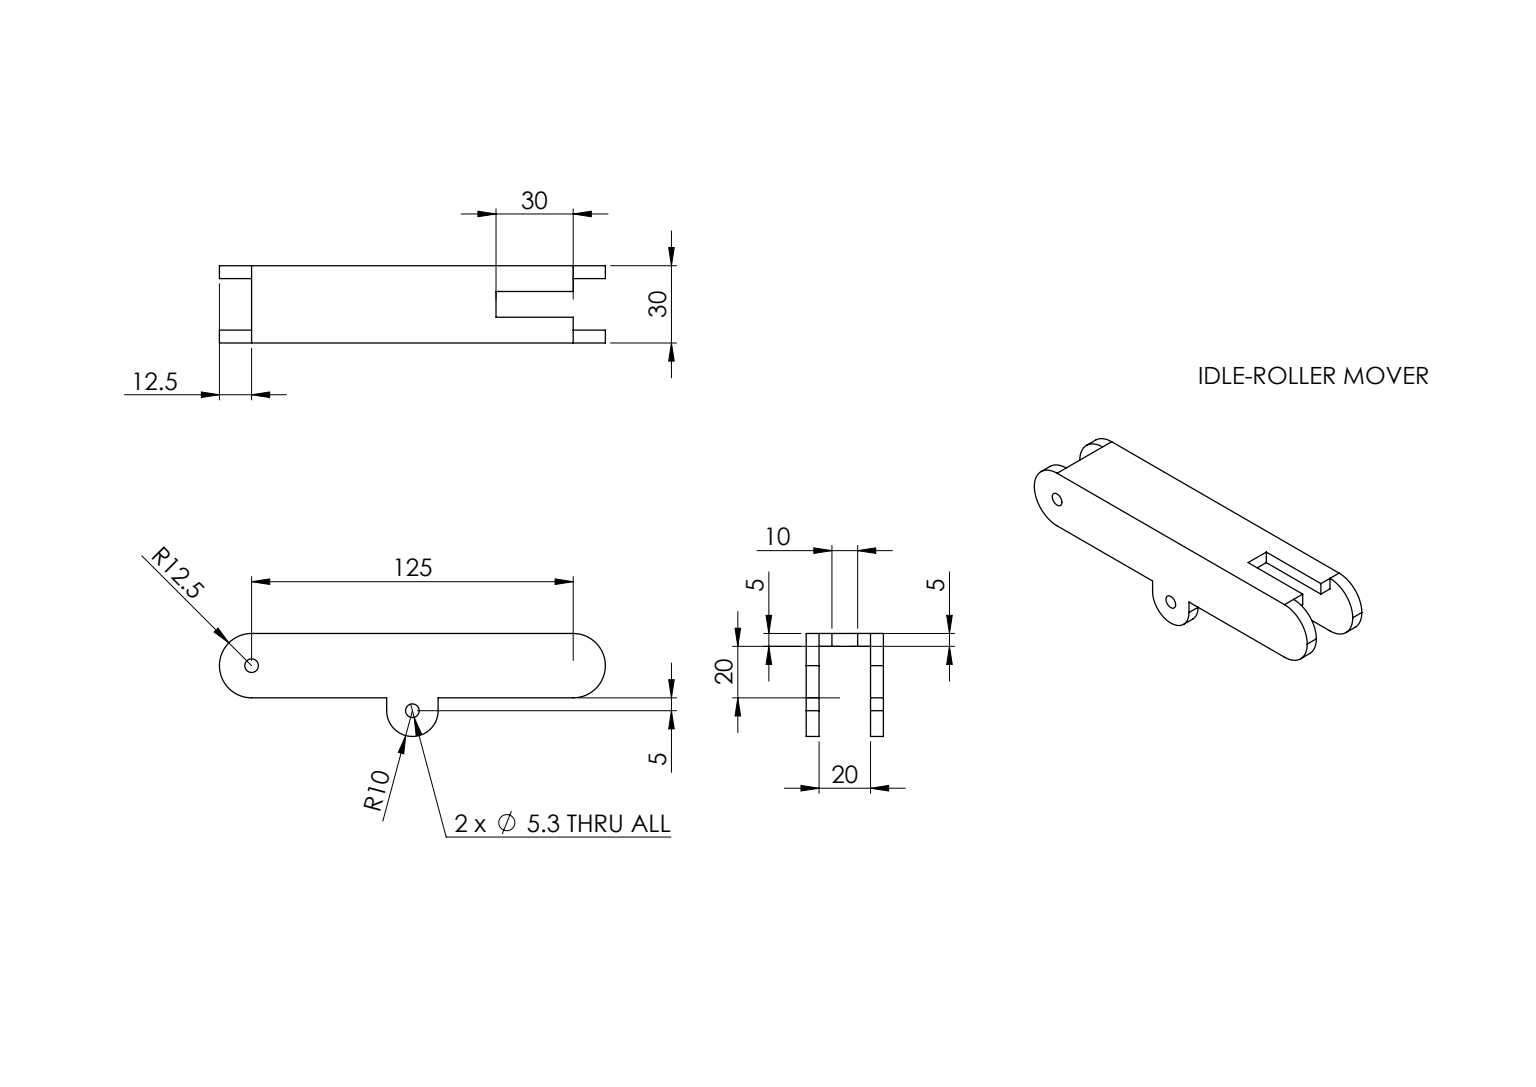
ISO-10303-21;
HEADER;
FILE_DESCRIPTION (('STEP AP214'),
    '1' );
FILE_NAME ('idle-roller mover.step',
    '2026-10-31T03:44:21',
    ( '' ),
    ( '' ),
    'SwSTEP 2.0',
    'SolidWorks 2026',
    '' );
FILE_SCHEMA (( 'AUTOMOTIVE_DESIGN' ));
ENDSEC;

DATA;
#62=VERTEX_POINT ( 'NONE', #14718 ) ;
#68=ADVANCED_FACE ( 'NONE', ( #1306 ), #2882, .T. ) ;
#78=CARTESIAN_POINT ( 'NONE',  ( -62.49999999999997158, 32.50000000000001421, 15.00000000000000000 ) ) ;
#85=LINE ( 'NONE', #5764, #17678 ) ;
#89=ORIENTED_EDGE ( 'NONE', *, *, #4960, .T. ) ;
#104=CARTESIAN_POINT ( 'NONE',  ( -62.49999999999997158, 32.50000000000001421, -15.00000000000000000 ) ) ;
#111=ORIENTED_EDGE ( 'NONE', *, *, #1854, .F. ) ;
#118=EDGE_CURVE ( 'NONE', #2113, #2665, #16595, .T. ) ;
#128=DIRECTION ( 'NONE',  ( 0.000000000000000000, -0.000000000000000000, 1.000000000000000000 ) ) ;
#164=VERTEX_POINT ( 'NONE', #8741 ) ;
#178=VERTEX_POINT ( 'NONE', #10980 ) ;
#180=ORIENTED_EDGE ( 'NONE', *, *, #9393, .F. ) ;
#211=DIRECTION ( 'NONE',  ( -0.000000000000000000, -0.000000000000000000, 1.000000000000000000 ) ) ;
#227=DIRECTION ( 'NONE',  ( 0.000000000000000000, -0.000000000000000000, 1.000000000000000000 ) ) ;
#232=EDGE_LOOP ( 'NONE', ( #13470, #855 ) ) ;
#236=PLANE ( 'NONE',  #7905 ) ;
#241=AXIS2_PLACEMENT_3D ( 'NONE', #17266, #3826, #15783 ) ;
#248=VERTEX_POINT ( 'NONE', #13911 ) ;
#260=CARTESIAN_POINT ( 'NONE',  ( 9.999999999999994671, 20.00000000000001421, -9.999999999999998224 ) ) ;
#273=VERTEX_POINT ( 'NONE', #10784 ) ;
#285=AXIS2_PLACEMENT_3D ( 'NONE', #12614, #3232, #18241 ) ;
#291=DIRECTION ( 'NONE',  ( 1.000000000000000000, 0.000000000000000000, 0.000000000000000000 ) ) ;
#304=FILL_AREA_STYLE_COLOUR ( '', #11512 ) ;
#308=CIRCLE ( 'NONE', #3740, 12.49999999999999645 ) ;
#311=DIRECTION ( 'NONE',  ( 1.000000000000000000, -0.000000000000000000, 0.000000000000000000 ) ) ;
#322=DIRECTION ( 'NONE',  ( 0.000000000000000000, 0.000000000000000000, -1.000000000000000000 ) ) ;
#342=FACE_OUTER_BOUND ( 'NONE', #4754, .T. ) ;
#350=AXIS2_PLACEMENT_3D ( 'NONE', #1219, #5627, #11312 ) ;
#355=DIRECTION ( 'NONE',  ( 0.000000000000000000, 0.000000000000000000, -1.000000000000000000 ) ) ;
#364=AXIS2_PLACEMENT_3D ( 'NONE', #11139, #15465, #17247 ) ;
#397=ORIENTED_EDGE ( 'NONE', *, *, #12870, .T. ) ;
#409=PLANE ( 'NONE',  #5457 ) ;
#418=AXIS2_PLACEMENT_3D ( 'NONE', #11692, #1217, #13364 ) ;
#474=DIRECTION ( 'NONE',  ( 0.000000000000000000, -0.000000000000000000, 1.000000000000000000 ) ) ;
#485=EDGE_LOOP ( 'NONE', ( #9928, #11888, #6922, #5916 ) ) ;
#487=SURFACE_SIDE_STYLE ('',( #18064 ) ) ;
#533=ORIENTED_EDGE ( 'NONE', *, *, #13929, .T. ) ;
#534=EDGE_CURVE ( 'NONE', #17889, #2561, #18649, .T. ) ;
#536=EDGE_CURVE ( 'NONE', #9835, #14591, #15254, .T. ) ;
#540=EDGE_CURVE ( 'NONE', #178, #11648, #7706, .T. ) ;
#563=ORIENTED_EDGE ( 'NONE', *, *, #9312, .F. ) ;
#574=STYLED_ITEM('',(#19461),#14815);
#579=MECHANICAL_DESIGN_GEOMETRIC_PRESENTATION_REPRESENTATION('',(#14012),#4333);
#599=VECTOR ( 'NONE', #11017, 1000.000000000000000 ) ;
#642=CIRCLE ( 'NONE', #6581, 9.999999999999998224 ) ;
#659=SHAPE_REPRESENTATION ( 'idle-roller mover', ( #10359 ), #7771 ) ;
#671=VERTEX_POINT ( 'NONE', #6520 ) ;
#674=FACE_OUTER_BOUND ( 'NONE', #12815, .T. ) ;
#680=CIRCLE ( 'NONE', #11624, 12.49999999999999645 ) ;
#699=PLANE ( 'NONE',  #16848 ) ;
#711=CYLINDRICAL_SURFACE ( 'NONE', #16596, 12.49999999999999645 ) ;
#768=CARTESIAN_POINT ( 'NONE',  ( 10.00000000000000000, 0.000000000000000000, 9.999999999999998224 ) ) ;
#770=DIRECTION ( 'NONE',  ( -0.000000000000000000, -0.000000000000000000, 1.000000000000000000 ) ) ;
#804=VECTOR ( 'NONE', #311, 1000.000000000000000 ) ;
#813=EDGE_CURVE ( 'NONE', #7075, #6422, #11344, .T. ) ;
#835=ORIENTED_EDGE ( 'NONE', *, *, #16599, .T. ) ;
#846=AXIS2_PLACEMENT_3D ( 'NONE', #4289, #19020, #14574 ) ;
#851=ORIENTED_EDGE ( 'NONE', *, *, #8320, .T. ) ;
#854=EDGE_LOOP ( 'NONE', ( #10763, #14737 ) ) ;
#855=ORIENTED_EDGE ( 'NONE', *, *, #534, .T. ) ;
#903=ADVANCED_FACE ( 'NONE', ( #342 ), #236, .F. ) ;
#904=DIRECTION ( 'NONE',  ( 1.000000000000000000, 0.000000000000000000, 0.000000000000000000 ) ) ;
#916=DIRECTION ( 'NONE',  ( -0.000000000000000000, 0.000000000000000000, -1.000000000000000000 ) ) ;
#933=VECTOR ( 'NONE', #904, 1000.000000000000000 ) ;
#946=CARTESIAN_POINT ( 'NONE',  ( -9.999999999999998224, 15.00000000000001776, -9.999999999999998224 ) ) ;
#969=LINE ( 'NONE', #768, #15487 ) ;
#970=CARTESIAN_POINT ( 'NONE',  ( 1.925929944387235853E-31, 15.00000000000001599, 9.999999999999998224 ) ) ;
#980=FACE_OUTER_BOUND ( 'NONE', #485, .T. ) ;
#981=LINE ( 'NONE', #18936, #3407 ) ;
#985=EDGE_LOOP ( 'NONE', ( #10470, #4595, #111, #14625 ) ) ;
#992=DIRECTION ( 'NONE',  ( 0.000000000000000000, 1.000000000000000000, 0.000000000000000000 ) ) ;
#1012=LINE ( 'NONE', #8840, #1882 ) ;
#1015=FACE_OUTER_BOUND ( 'NONE', #18810, .T. ) ;
#1027=ORIENTED_EDGE ( 'NONE', *, *, #13929, .F. ) ;
#1062=CARTESIAN_POINT ( 'NONE',  ( 32.49999999999998579, 40.00000000000001421, 15.00000000000000000 ) ) ;
#1103=DIRECTION ( 'NONE',  ( 0.000000000000000000, 0.000000000000000000, -1.000000000000000000 ) ) ;
#1116=ORIENTED_EDGE ( 'NONE', *, *, #536, .T. ) ;
#1125=DIRECTION ( 'NONE',  ( -0.000000000000000000, -0.000000000000000000, 1.000000000000000000 ) ) ;
#1149=ORIENTED_EDGE ( 'NONE', *, *, #15610, .T. ) ;
#1184=DIRECTION ( 'NONE',  ( 1.000000000000000000, 0.000000000000000000, 0.000000000000000000 ) ) ;
#1203=DIRECTION ( 'NONE',  ( 0.000000000000000000, 0.000000000000000000, -1.000000000000000000 ) ) ;
#1217=DIRECTION ( 'NONE',  ( 0.000000000000000000, 1.000000000000000000, 0.000000000000000000 ) ) ;
#1219=CARTESIAN_POINT ( 'NONE',  ( -62.49999999999997158, 32.50000000000001421, -9.999999999999998224 ) ) ;
#1239=ORIENTED_EDGE ( 'NONE', *, *, #7238, .T. ) ;
#1247=VERTEX_POINT ( 'NONE', #18585 ) ;
#1281=CARTESIAN_POINT ( 'NONE',  ( -62.49999999999997158, 32.50000000000001421, 9.999999999999998224 ) ) ;
#1298=ORIENTED_EDGE ( 'NONE', *, *, #536, .F. ) ;
#1303=AXIS2_PLACEMENT_3D ( 'NONE', #18296, #7784, #10909 ) ;
#1306=FACE_OUTER_BOUND ( 'NONE', #16945, .T. ) ;
#1315=VECTOR ( 'NONE', #1680, 1000.000000000000000 ) ;
#1349=CARTESIAN_POINT ( 'NONE',  ( -62.49999999999997158, 20.00000000000001421, -15.00000000000000000 ) ) ;
#1351=LINE ( 'NONE', #1062, #18417 ) ;
#1353=CARTESIAN_POINT ( 'NONE',  ( 32.49999999999998579, 45.00000000000001421, 5.000000000000003553 ) ) ;
#1359=PRODUCT_DEFINITION ( 'UNKNOWN', '', #1975, #10856 ) ;
#1381=VECTOR ( 'NONE', #19322, 1000.000000000000000 ) ;
#1404=CARTESIAN_POINT ( 'NONE',  ( -74.99999999999997158, 32.50000000000001421, -15.00000000000000000 ) ) ;
#1452=CARTESIAN_POINT ( 'NONE',  ( 32.49999999999998579, 5.000000000000018652, -4.999999999999996447 ) ) ;
#1457=FACE_OUTER_BOUND ( 'NONE', #9301, .T. ) ;
#1462=VERTEX_POINT ( 'NONE', #18073 ) ;
#1485=CARTESIAN_POINT ( 'NONE',  ( -62.49999999999997158, 32.50000000000001421, -15.00000000000000000 ) ) ;
#1487=DIRECTION ( 'NONE',  ( 1.000000000000000000, 0.000000000000000000, 0.000000000000000000 ) ) ;
#1488=ADVANCED_FACE ( 'NONE', ( #2972 ), #16696, .T. ) ;
#1518=VECTOR ( 'NONE', #17948, 1000.000000000000000 ) ;
#1530=DIRECTION ( 'NONE',  ( 0.000000000000000000, 0.000000000000000000, -1.000000000000000000 ) ) ;
#1567=AXIS2_PLACEMENT_3D ( 'NONE', #6482, #12664, #14320 ) ;
#1594=AXIS2_PLACEMENT_3D ( 'NONE', #7740, #4809, #4899 ) ;
#1613=ADVANCED_FACE ( 'NONE', ( #13831 ), #12652, .F. ) ;
#1614=EDGE_CURVE ( 'NONE', #10922, #10528, #6471, .T. ) ;
#1617=DIRECTION ( 'NONE',  ( 0.000000000000000000, 0.000000000000000000, -1.000000000000000000 ) ) ;
#1618=ADVANCED_FACE ( 'NONE', ( #9596, #12451, #10883 ), #2072, .F. ) ;
#1621=CARTESIAN_POINT ( 'NONE',  ( -62.49999999999997158, 20.00000000000001421, -15.00000000000000000 ) ) ;
#1623=FACE_OUTER_BOUND ( 'NONE', #18650, .T. ) ;
#1674=ORIENTED_EDGE ( 'NONE', *, *, #15749, .F. ) ;
#1680=DIRECTION ( 'NONE',  ( 1.000000000000000000, -0.000000000000000000, 0.000000000000000000 ) ) ;
#1682=DIRECTION ( 'NONE',  ( -0.000000000000000000, -0.000000000000000000, 1.000000000000000000 ) ) ;
#1705=ORIENTED_EDGE ( 'NONE', *, *, #3062, .F. ) ;
#1721=ADVANCED_FACE ( 'NONE', ( #15306 ), #699, .F. ) ;
#1724=ORIENTED_EDGE ( 'NONE', *, *, #17366, .F. ) ;
#1739=CYLINDRICAL_SURFACE ( 'NONE', #17926, 12.49999999999999645 ) ;
#1780=EDGE_CURVE ( 'NONE', #9457, #2897, #16089, .T. ) ;
#1825=CARTESIAN_POINT ( 'NONE',  ( 62.49999999999998579, 45.00000000000001421, -9.999999999999998224 ) ) ;
#1854=EDGE_CURVE ( 'NONE', #7017, #7129, #17757, .T. ) ;
#1882=VECTOR ( 'NONE', #5606, 1000.000000000000000 ) ;
#1900=CIRCLE ( 'NONE', #12847, 12.49999999999999645 ) ;
#1955=ORIENTED_EDGE ( 'NONE', *, *, #11365, .T. ) ;
#1970=EDGE_CURVE ( 'NONE', #17741, #6607, #4613, .T. ) ;
#1975=PRODUCT_DEFINITION_FORMATION_WITH_SPECIFIED_SOURCE ( 'ANY', '', #10075, .NOT_KNOWN. ) ;
#2016=LINE ( 'NONE', #10822, #5296 ) ;
#2022=ORIENTED_EDGE ( 'NONE', *, *, #11676, .F. ) ;
#2028=CARTESIAN_POINT ( 'NONE',  ( 0.000000000000000000, 20.00000000000001421, -9.999999999999998224 ) ) ;
#2042=CYLINDRICAL_SURFACE ( 'NONE', #285, 2.649999999999988365 ) ;
#2071=LINE ( 'NONE', #16695, #13282 ) ;
#2072=PLANE ( 'NONE',  #12758 ) ;
#2079=DIRECTION ( 'NONE',  ( -1.000000000000000000, 0.000000000000000000, 1.224646799147353207E-16 ) ) ;
#2103=LINE ( 'NONE', #15724, #17590 ) ;
#2112=DIRECTION ( 'NONE',  ( -0.000000000000000000, 1.000000000000000000, -0.000000000000000000 ) ) ;
#2113=VERTEX_POINT ( 'NONE', #13896 ) ;
#2121=CIRCLE ( 'NONE', #8046, 2.649999999999985700 ) ;
#2133=ORIENTED_EDGE ( 'NONE', *, *, #13598, .F. ) ;
#2134=FACE_OUTER_BOUND ( 'NONE', #12540, .T. ) ;
#2136=VECTOR ( 'NONE', #2285, 1000.000000000000000 ) ;
#2137=EDGE_CURVE ( 'NONE', #3410, #5817, #10817, .T. ) ;
#2143=ORIENTED_EDGE ( 'NONE', *, *, #17441, .F. ) ;
#2192=VERTEX_POINT ( 'NONE', #14487 ) ;
#2213=DIRECTION ( 'NONE',  ( 0.000000000000000000, 0.000000000000000000, -1.000000000000000000 ) ) ;
#2214=ORIENTED_EDGE ( 'NONE', *, *, #15651, .T. ) ;
#2217=EDGE_CURVE ( 'NONE', #62, #18826, #7388, .T. ) ;
#2230=ADVANCED_FACE ( 'NONE', ( #13018 ), #14284, .T. ) ;
#2240=ORIENTED_EDGE ( 'NONE', *, *, #11403, .T. ) ;
#2272=DIRECTION ( 'NONE',  ( -0.000000000000000000, -0.000000000000000000, -1.000000000000000000 ) ) ;
#2285=DIRECTION ( 'NONE',  ( -0.000000000000000000, -0.000000000000000000, -1.000000000000000000 ) ) ;
#2311=ORIENTED_EDGE ( 'NONE', *, *, #1970, .T. ) ;
#2356=DIRECTION ( 'NONE',  ( 1.000000000000000000, 0.000000000000000000, 0.000000000000000000 ) ) ;
#2358=ORIENTED_EDGE ( 'NONE', *, *, #6658, .T. ) ;
#2373=CARTESIAN_POINT ( 'NONE',  ( 2.649999999999987477, 15.00000000000001599, 15.00000000000000178 ) ) ;
#2377=CARTESIAN_POINT ( 'NONE',  ( 10.00000000000000000, 15.00000000000001776, 15.00000000000000000 ) ) ;
#2414=VECTOR ( 'NONE', #13659, 1000.000000000000000 ) ;
#2433=VERTEX_POINT ( 'NONE', #3860 ) ;
#2437=VECTOR ( 'NONE', #17878, 1000.000000000000000 ) ;
#2454=EDGE_CURVE ( 'NONE', #2113, #6630, #5693, .T. ) ;
#2457=ORIENTED_EDGE ( 'NONE', *, *, #3348, .T. ) ;
#2459=DIRECTION ( 'NONE',  ( -0.000000000000000000, -0.000000000000000000, 1.000000000000000000 ) ) ;
#2548=CIRCLE ( 'NONE', #17575, 12.49999999999999645 ) ;
#2559=AXIS2_PLACEMENT_3D ( 'NONE', #1281, #8422, #19338 ) ;
#2561=VERTEX_POINT ( 'NONE', #17689 ) ;
#2587=LINE ( 'NONE', #14415, #2136 ) ;
#2620=CARTESIAN_POINT ( 'NONE',  ( 75.00000000000000000, 32.50000000000001421, 15.00000000000000000 ) ) ;
#2633=ADVANCED_FACE ( 'NONE', ( #8354 ), #5512, .T. ) ;
#2642=ORIENTED_EDGE ( 'NONE', *, *, #118, .F. ) ;
#2646=CARTESIAN_POINT ( 'NONE',  ( -62.49999999999997158, 32.50000000000001421, 15.00000000000000000 ) ) ;
#2665=VERTEX_POINT ( 'NONE', #1404 ) ;
#2685=DIRECTION ( 'NONE',  ( 1.000000000000000000, 0.000000000000000000, -0.000000000000000000 ) ) ;
#2723=EDGE_CURVE ( 'NONE', #1247, #2192, #18742, .T. ) ;
#2725=DIRECTION ( 'NONE',  ( -1.000000000000000000, 0.000000000000000000, 1.224646799147353207E-16 ) ) ;
#2802=VERTEX_POINT ( 'NONE', #12743 ) ;
#2812=CIRCLE ( 'NONE', #13129, 12.49999999999999645 ) ;
#2814=AXIS2_PLACEMENT_3D ( 'NONE', #12299, #355, #16535 ) ;
#2825=EDGE_CURVE ( 'NONE', #8729, #6112, #16066, .T. ) ;
#2830=ORIENTED_EDGE ( 'NONE', *, *, #4507, .T. ) ;
#2859=AXIS2_PLACEMENT_3D ( 'NONE', #19237, #5483, #7155 ) ;
#2871=CARTESIAN_POINT ( 'NONE',  ( 0.000000000000000000, 0.000000000000000000, 0.000000000000000000 ) ) ;
#2882=CYLINDRICAL_SURFACE ( 'NONE', #11472, 12.49999999999999645 ) ;
#2895=EDGE_LOOP ( 'NONE', ( #13031, #2901 ) ) ;
#2897=VERTEX_POINT ( 'NONE', #260 ) ;
#2901=ORIENTED_EDGE ( 'NONE', *, *, #17364, .F. ) ;
#2913=AXIS2_PLACEMENT_3D ( 'NONE', #17621, #11508, #17325 ) ;
#2914=ORIENTED_EDGE ( 'NONE', *, *, #9264, .T. ) ;
#2922=ORIENTED_EDGE ( 'NONE', *, *, #15885, .T. ) ;
#2932=CARTESIAN_POINT ( 'NONE',  ( 75.00000000000000000, 32.50000000000001421, -15.00000000000000000 ) ) ;
#2933=ORIENTED_EDGE ( 'NONE', *, *, #11365, .F. ) ;
#2937=CARTESIAN_POINT ( 'NONE',  ( 62.49999999999998579, 45.00000000000001421, 9.999999999999998224 ) ) ;
#2957=EDGE_CURVE ( 'NONE', #2433, #6630, #8982, .T. ) ;
#2967=VECTOR ( 'NONE', #17100, 1000.000000000000000 ) ;
#2972=FACE_OUTER_BOUND ( 'NONE', #17073, .T. ) ;
#2981=ORIENTED_EDGE ( 'NONE', *, *, #7617, .T. ) ;
#2982=ADVANCED_FACE ( 'NONE', ( #15072 ), #1739, .T. ) ;
#3012=ORIENTED_EDGE ( 'NONE', *, *, #6302, .F. ) ;
#3055=EDGE_CURVE ( 'NONE', #19088, #6925, #8275, .T. ) ;
#3062=EDGE_CURVE ( 'NONE', #10814, #11786, #3397, .T. ) ;
#3066=DIRECTION ( 'NONE',  ( 1.000000000000000000, -0.000000000000000000, 0.000000000000000000 ) ) ;
#3077=CARTESIAN_POINT ( 'NONE',  ( -62.49999999999997158, 32.50000000000001421, -15.00000000000000000 ) ) ;
#3090=DIRECTION ( 'NONE',  ( 1.000000000000000000, 0.000000000000000000, 0.000000000000000000 ) ) ;
#3140=CIRCLE ( 'NONE', #16292, 2.649999999999987477 ) ;
#3158=CARTESIAN_POINT ( 'NONE',  ( -2.649999999999987477, 15.00000000000001599, 15.00000000000000178 ) ) ;
#3164=DIRECTION ( 'NONE',  ( 1.000000000000000000, 0.000000000000000000, 0.000000000000000000 ) ) ;
#3170=AXIS2_PLACEMENT_3D ( 'NONE', #18983, #12788, #8571 ) ;
#3192=CARTESIAN_POINT ( 'NONE',  ( -62.49999999999997158, 45.00000000000001421, 15.00000000000000000 ) ) ;
#3193=LINE ( 'NONE', #5830, #8882 ) ;
#3232=DIRECTION ( 'NONE',  ( -0.000000000000000000, -0.000000000000000000, 1.000000000000000000 ) ) ;
#3256=CARTESIAN_POINT ( 'NONE',  ( 62.49999999999998579, 40.00000000000001421, 9.999999999999998224 ) ) ;
#3272=ORIENTED_EDGE ( 'NONE', *, *, #10957, .T. ) ;
#3287=ORIENTED_EDGE ( 'NONE', *, *, #17366, .T. ) ;
#3294=CARTESIAN_POINT ( 'NONE',  ( 32.49999999999998579, 5.000000000000018652, 5.000000000000003553 ) ) ;
#3307=EDGE_CURVE ( 'NONE', #5263, #6112, #12645, .T. ) ;
#3322=LINE ( 'NONE', #3602, #15614 ) ;
#3323=ORIENTED_EDGE ( 'NONE', *, *, #17364, .T. ) ;
#3328=ORIENTED_EDGE ( 'NONE', *, *, #12262, .F. ) ;
#3337=DIRECTION ( 'NONE',  ( -0.000000000000000000, -0.000000000000000000, 1.000000000000000000 ) ) ;
#3342=ORIENTED_EDGE ( 'NONE', *, *, #17496, .T. ) ;
#3343=( NAMED_UNIT ( * ) PLANE_ANGLE_UNIT ( ) SI_UNIT ( $, .RADIAN. ) );
#3348=EDGE_CURVE ( 'NONE', #7873, #4201, #3193, .T. ) ;
#3355=DIRECTION ( 'NONE',  ( 0.000000000000000000, 0.000000000000000000, -1.000000000000000000 ) ) ;
#3381=FACE_OUTER_BOUND ( 'NONE', #7891, .T. ) ;
#3386=DIRECTION ( 'NONE',  ( -0.000000000000000000, -0.000000000000000000, 1.000000000000000000 ) ) ;
#3397=LINE ( 'NONE', #2028, #17988 ) ;
#3407=VECTOR ( 'NONE', #11356, 1000.000000000000000 ) ;
#3410=VERTEX_POINT ( 'NONE', #9155 ) ;
#3437=ORIENTED_EDGE ( 'NONE', *, *, #2137, .T. ) ;
#3441=ORIENTED_EDGE ( 'NONE', *, *, #6041, .T. ) ;
#3452=DIRECTION ( 'NONE',  ( 0.000000000000000000, 0.000000000000000000, 1.000000000000000000 ) ) ;
#3465=CIRCLE ( 'NONE', #4729, 2.649999999999988809 ) ;
#3482=LINE ( 'NONE', #7972, #7826 ) ;
#3506=CARTESIAN_POINT ( 'NONE',  ( 75.00000000000000000, 32.50000000000001421, 15.00000000000000000 ) ) ;
#3509=DIRECTION ( 'NONE',  ( 0.000000000000000000, 0.000000000000000000, -1.000000000000000000 ) ) ;
#3516=DIRECTION ( 'NONE',  ( -0.000000000000000000, 0.000000000000000000, -1.000000000000000000 ) ) ;
#3527=ORIENTED_EDGE ( 'NONE', *, *, #2217, .F. ) ;
#3554=CARTESIAN_POINT ( 'NONE',  ( 62.50000000000000000, 32.50000000000001421, 15.00000000000000000 ) ) ;
#3565=CARTESIAN_POINT ( 'NONE',  ( 62.49999999999998579, 45.00000000000001421, 15.00000000000000000 ) ) ;
#3582=EDGE_CURVE ( 'NONE', #15125, #273, #11092, .T. ) ;
#3586=ORIENTED_EDGE ( 'NONE', *, *, #4960, .F. ) ;
#3602=CARTESIAN_POINT ( 'NONE',  ( 9.999999999999994671, 20.00000000000001421, 15.00000000000000000 ) ) ;
#3613=LINE ( 'NONE', #7829, #15804 ) ;
#3644=DIRECTION ( 'NONE',  ( -0.000000000000000000, -0.000000000000000000, 1.000000000000000000 ) ) ;
#3648=EDGE_CURVE ( 'NONE', #10516, #8542, #18674, .T. ) ;
#3659=ADVANCED_FACE ( 'NONE', ( #16110, #18872, #1015 ), #10200, .F. ) ;
#3673=CARTESIAN_POINT ( 'NONE',  ( -62.49999999999997158, 32.50000000000001421, 15.00000000000000000 ) ) ;
#3675=DIRECTION ( 'NONE',  ( -0.000000000000000000, -0.000000000000000000, 1.000000000000000000 ) ) ;
#3700=AXIS2_PLACEMENT_3D ( 'NONE', #12562, #3644, #18372 ) ;
#3705=CARTESIAN_POINT ( 'NONE',  ( 62.49999999999998579, 20.00000000000001421, 15.00000000000000000 ) ) ;
#3708=VERTEX_POINT ( 'NONE', #12869 ) ;
#3715=DIRECTION ( 'NONE',  ( -1.224646799147353207E-16, 0.000000000000000000, -1.000000000000000000 ) ) ;
#3740=AXIS2_PLACEMENT_3D ( 'NONE', #11015, #2213, #17022 ) ;
#3763=CARTESIAN_POINT ( 'NONE',  ( 1.925929944387235853E-31, 15.00000000000001599, 15.00000000000000000 ) ) ;
#3771=VERTEX_POINT ( 'NONE', #19172 ) ;
#3774=ADVANCED_FACE ( 'NONE', ( #17297 ), #9815, .T. ) ;
#3796=DIRECTION ( 'NONE',  ( -1.000000000000000000, 0.000000000000000000, 0.000000000000000000 ) ) ;
#3799=ORIENTED_EDGE ( 'NONE', *, *, #16660, .T. ) ;
#3800=DIRECTION ( 'NONE',  ( -1.000000000000000000, 0.000000000000000000, -0.000000000000000000 ) ) ;
#3818=DIRECTION ( 'NONE',  ( 1.000000000000000000, 0.000000000000000000, 0.000000000000000000 ) ) ;
#3826=DIRECTION ( 'NONE',  ( -0.000000000000000000, -0.000000000000000000, 1.000000000000000000 ) ) ;
#3860=CARTESIAN_POINT ( 'NONE',  ( -62.49999999999997158, 40.00000000000001421, -9.999999999999998224 ) ) ;
#3896=EDGE_LOOP ( 'NONE', ( #7677, #3272, #11341, #7131 ) ) ;
#3907=EDGE_LOOP ( 'NONE', ( #12635, #19029, #3342, #11438 ) ) ;
#3914=LINE ( 'NONE', #8307, #7534 ) ;
#3939=LINE ( 'NONE', #17477, #5569 ) ;
#3959=FACE_OUTER_BOUND ( 'NONE', #13204, .T. ) ;
#3989=ORIENTED_EDGE ( 'NONE', *, *, #540, .T. ) ;
#3993=ORIENTED_EDGE ( 'NONE', *, *, #9285, .F. ) ;
#4003=ADVANCED_FACE ( 'NONE', ( #4635 ), #409, .F. ) ;
#4013=LINE ( 'NONE', #15216, #14946 ) ;
#4028=LINE ( 'NONE', #9891, #9519 ) ;
#4036=DIRECTION ( 'NONE',  ( -0.000000000000000000, 0.000000000000000000, -1.000000000000000000 ) ) ;
#4070=ORIENTED_EDGE ( 'NONE', *, *, #7617, .F. ) ;
#4083=CARTESIAN_POINT ( 'NONE',  ( 1.925929944387235853E-31, 15.00000000000001599, -9.999999999999998224 ) ) ;
#4086=ORIENTED_EDGE ( 'NONE', *, *, #7359, .F. ) ;
#4102=CARTESIAN_POINT ( 'NONE',  ( -9.999999999999996447, 25.00000000000001776, 15.00000000000000000 ) ) ;
#4133=EDGE_CURVE ( 'NONE', #13670, #1462, #2071, .T. ) ;
#4136=( NAMED_UNIT ( * ) PLANE_ANGLE_UNIT ( ) SI_UNIT ( $, .RADIAN. ) );
#4139=ORIENTED_EDGE ( 'NONE', *, *, #5848, .T. ) ;
#4162=FACE_OUTER_BOUND ( 'NONE', #4530, .T. ) ;
#4163=ORIENTED_EDGE ( 'NONE', *, *, #6041, .F. ) ;
#4179=VERTEX_POINT ( 'NONE', #9797 ) ;
#4195=PLANE ( 'NONE',  #6785 ) ;
#4201=VERTEX_POINT ( 'NONE', #15890 ) ;
#4237=EDGE_CURVE ( 'NONE', #248, #17308, #4028, .T. ) ;
#4247=ADVANCED_FACE ( 'NONE', ( #11558 ), #11458, .F. ) ;
#4248=VERTEX_POINT ( 'NONE', #2373 ) ;
#4262=CARTESIAN_POINT ( 'NONE',  ( 62.50000000000000000, 32.50000000000001421, -9.999999999999998224 ) ) ;
#4280=ORIENTED_EDGE ( 'NONE', *, *, #18031, .F. ) ;
#4289=CARTESIAN_POINT ( 'NONE',  ( -62.49999999999997158, 32.50000000000001421, 15.00000000000000000 ) ) ;
#4333=( GEOMETRIC_REPRESENTATION_CONTEXT ( 3 ) GLOBAL_UNCERTAINTY_ASSIGNED_CONTEXT ( ( #7345 ) ) GLOBAL_UNIT_ASSIGNED_CONTEXT ( ( #10583, #15004, #13903 ) ) REPRESENTATION_CONTEXT ( 'NONE', 'WORKASPACE' ) );
#4358=LINE ( 'NONE', #3192, #4605 ) ;
#4377=DIRECTION ( 'NONE',  ( -1.000000000000000000, 0.000000000000000000, 0.000000000000000000 ) ) ;
#4388=CIRCLE ( 'NONE', #14066, 12.49999999999999645 ) ;
#4393=DIRECTION ( 'NONE',  ( -0.000000000000000000, 0.000000000000000000, -1.000000000000000000 ) ) ;
#4438=CIRCLE ( 'NONE', #16334, 2.649999999999985700 ) ;
#4463=DIRECTION ( 'NONE',  ( -0.000000000000000000, -0.000000000000000000, 1.000000000000000000 ) ) ;
#4477=EDGE_CURVE ( 'NONE', #10516, #7873, #13293, .T. ) ;
#4487=CARTESIAN_POINT ( 'NONE',  ( 2.649999999999988365, 15.00000000000001599, 15.00000000000000000 ) ) ;
#4497=DIRECTION ( 'NONE',  ( 0.000000000000000000, 0.000000000000000000, -1.000000000000000000 ) ) ;
#4501=ORIENTED_EDGE ( 'NONE', *, *, #2957, .F. ) ;
#4502=ORIENTED_EDGE ( 'NONE', *, *, #18699, .T. ) ;
#4507=EDGE_CURVE ( 'NONE', #1247, #17702, #3613, .T. ) ;
#4513=VERTEX_POINT ( 'NONE', #6449 ) ;
#4530=EDGE_LOOP ( 'NONE', ( #7481, #5283, #8817, #3012 ) ) ;
#4532=AXIS2_PLACEMENT_3D ( 'NONE', #15814, #6878, #17392 ) ;
#4555=ORIENTED_EDGE ( 'NONE', *, *, #2825, .T. ) ;
#4568=FACE_OUTER_BOUND ( 'NONE', #16154, .T. ) ;
#4587=VECTOR ( 'NONE', #16481, 1000.000000000000000 ) ;
#4595=ORIENTED_EDGE ( 'NONE', *, *, #10584, .T. ) ;
#4605=VECTOR ( 'NONE', #4463, 1000.000000000000000 ) ;
#4608=CARTESIAN_POINT ( 'NONE',  ( -59.84999999999998721, 32.50000000000001421, -15.00000000000000000 ) ) ;
#4613=LINE ( 'NONE', #13324, #19332 ) ;
#4623=PRESENTATION_STYLE_ASSIGNMENT (( #18355 ) ) ;
#4628=DIRECTION ( 'NONE',  ( 1.000000000000000000, 0.000000000000000000, -0.000000000000000000 ) ) ;
#4635=FACE_OUTER_BOUND ( 'NONE', #19090, .T. ) ;
#4644=FACE_OUTER_BOUND ( 'NONE', #10586, .T. ) ;
#4649=ORIENTED_EDGE ( 'NONE', *, *, #14215, .F. ) ;
#4673=AXIS2_PLACEMENT_3D ( 'NONE', #11228, #6632, #3800 ) ;
#4680=EDGE_CURVE ( 'NONE', #9490, #11811, #969, .T. ) ;
#4693=DIRECTION ( 'NONE',  ( 0.000000000000000000, 0.000000000000000000, -1.000000000000000000 ) ) ;
#4715=DIRECTION ( 'NONE',  ( 0.000000000000000000, -1.000000000000000000, 0.000000000000000000 ) ) ;
#4729=AXIS2_PLACEMENT_3D ( 'NONE', #8218, #770, #3818 ) ;
#4753=LINE ( 'NONE', #1621, #18397 ) ;
#4754=EDGE_LOOP ( 'NONE', ( #15836, #9958, #6897, #17122, #11407, #9667, #563, #15561 ) ) ;
#4809=DIRECTION ( 'NONE',  ( 1.000000000000000000, 0.000000000000000000, -0.000000000000000000 ) ) ;
#4816=ORIENTED_EDGE ( 'NONE', *, *, #3307, .T. ) ;
#4851=CARTESIAN_POINT ( 'NONE',  ( 62.49999999999998579, 45.00000000000001421, -15.00000000000000000 ) ) ;
#4870=DIRECTION ( 'NONE',  ( 0.000000000000000000, -0.000000000000000000, 1.000000000000000000 ) ) ;
#4886=ORIENTED_EDGE ( 'NONE', *, *, #14851, .F. ) ;
#4893=PLANE ( 'NONE',  #15064 ) ;
#4897=EDGE_CURVE ( 'NONE', #6925, #18236, #19123, .T. ) ;
#4899=DIRECTION ( 'NONE',  ( -0.000000000000000000, 0.000000000000000000, -1.000000000000000000 ) ) ;
#4939=DIRECTION ( 'NONE',  ( -0.000000000000000000, 1.000000000000000000, -0.000000000000000000 ) ) ;
#4960=EDGE_CURVE ( 'NONE', #3410, #1462, #85, .T. ) ;
#4974=EDGE_CURVE ( 'NONE', #4179, #18236, #14773, .T. ) ;
#4989=ORIENTED_EDGE ( 'NONE', *, *, #5848, .F. ) ;
#4993=VECTOR ( 'NONE', #8123, 1000.000000000000000 ) ;
#4999=ORIENTED_EDGE ( 'NONE', *, *, #813, .T. ) ;
#5018=VECTOR ( 'NONE', #3066, 1000.000000000000000 ) ;
#5025=LINE ( 'NONE', #18579, #12193 ) ;
#5052=VECTOR ( 'NONE', #7700, 1000.000000000000000 ) ;
#5065=ORIENTED_EDGE ( 'NONE', *, *, #2454, .F. ) ;
#5079=ORIENTED_EDGE ( 'NONE', *, *, #15036, .T. ) ;
#5093=ORIENTED_EDGE ( 'NONE', *, *, #13389, .T. ) ;
#5101=EDGE_LOOP ( 'NONE', ( #17348, #1149, #5819, #12911 ) ) ;
#5122=EDGE_CURVE ( 'NONE', #10528, #7075, #13939, .T. ) ;
#5129=AXIS2_PLACEMENT_3D ( 'NONE', #4262, #7200, #16228 ) ;
#5131=CYLINDRICAL_SURFACE ( 'NONE', #13160, 2.649999999999988365 ) ;
#5169=CARTESIAN_POINT ( 'NONE',  ( -9.999999999999994671, 20.00000000000001421, 15.00000000000000000 ) ) ;
#5178=ORIENTED_EDGE ( 'NONE', *, *, #7458, .F. ) ;
#5196=CARTESIAN_POINT ( 'NONE',  ( 0.000000000000000000, 0.000000000000000000, 15.00000000000000000 ) ) ;
#5217=CARTESIAN_POINT ( 'NONE',  ( -65.14999999999996305, 32.50000000000001421, 15.00000000000000000 ) ) ;
#5234=CYLINDRICAL_SURFACE ( 'NONE', #3170, 12.49999999999999645 ) ;
#5257=FACE_BOUND ( 'NONE', #15200, .T. ) ;
#5263=VERTEX_POINT ( 'NONE', #14330 ) ;
#5269=ORIENTED_EDGE ( 'NONE', *, *, #11074, .F. ) ;
#5277=CARTESIAN_POINT ( 'NONE',  ( -9.999999999999998224, 15.00000000000001776, -15.00000000000000000 ) ) ;
#5283=ORIENTED_EDGE ( 'NONE', *, *, #11074, .T. ) ;
#5284=CARTESIAN_POINT ( 'NONE',  ( 10.00000000000000000, 15.00000000000001776, -9.999999999999998224 ) ) ;
#5292=DIRECTION ( 'NONE',  ( 0.000000000000000000, 1.000000000000000000, 0.000000000000000000 ) ) ;
#5296=VECTOR ( 'NONE', #3386, 1000.000000000000000 ) ;
#5309=AXIS2_PLACEMENT_3D ( 'NONE', #7070, #2685, #16007 ) ;
#5310=EDGE_CURVE ( 'NONE', #2665, #12330, #11072, .T. ) ;
#5312=DIRECTION ( 'NONE',  ( -1.000000000000000000, 0.000000000000000000, 1.224646799147353207E-16 ) ) ;
#5332=CIRCLE ( 'NONE', #10334, 2.649999999999988365 ) ;
#5366=ORIENTED_EDGE ( 'NONE', *, *, #17787, .T. ) ;
#5370=ORIENTED_EDGE ( 'NONE', *, *, #14851, .T. ) ;
#5418=DIRECTION ( 'NONE',  ( 1.000000000000000000, 0.000000000000000000, 0.000000000000000000 ) ) ;
#5452=EDGE_CURVE ( 'NONE', #248, #2665, #8504, .T. ) ;
#5456=ORIENTED_EDGE ( 'NONE', *, *, #4974, .T. ) ;
#5457=AXIS2_PLACEMENT_3D ( 'NONE', #14112, #18364, #10785 ) ;
#5483=DIRECTION ( 'NONE',  ( -0.000000000000000000, -0.000000000000000000, 1.000000000000000000 ) ) ;
#5487=DIRECTION ( 'NONE',  ( 0.000000000000000000, -0.000000000000000000, 1.000000000000000000 ) ) ;
#5501=PLANE ( 'NONE',  #5309 ) ;
#5512=CYLINDRICAL_SURFACE ( 'NONE', #18865, 12.49999999999999645 ) ;
#5515=CARTESIAN_POINT ( 'NONE',  ( -2.649999999999988365, 15.00000000000001599, 9.999999999999998224 ) ) ;
#5569=VECTOR ( 'NONE', #4036, 1000.000000000000000 ) ;
#5606=DIRECTION ( 'NONE',  ( -0.000000000000000000, -0.000000000000000000, 1.000000000000000000 ) ) ;
#5608=ORIENTED_EDGE ( 'NONE', *, *, #17496, .F. ) ;
#5627=DIRECTION ( 'NONE',  ( 0.000000000000000000, 0.000000000000000000, -1.000000000000000000 ) ) ;
#5654=CIRCLE ( 'NONE', #2559, 2.649999999999985700 ) ;
#5663=DIRECTION ( 'NONE',  ( 1.000000000000000000, 0.000000000000000000, -0.000000000000000000 ) ) ;
#5693=CIRCLE ( 'NONE', #10693, 12.49999999999999645 ) ;
#5711=CARTESIAN_POINT ( 'NONE',  ( 9.999999999999994671, 20.00000000000001421, -15.00000000000000000 ) ) ;
#5732=CYLINDRICAL_SURFACE ( 'NONE', #15564, 2.649999999999985700 ) ;
#5764=CARTESIAN_POINT ( 'NONE',  ( -9.999999999999998224, 15.00000000000001776, 15.00000000000000000 ) ) ;
#5773=CYLINDRICAL_SURFACE ( 'NONE', #241, 2.649999999999985700 ) ;
#5776=ORIENTED_EDGE ( 'NONE', *, *, #12870, .F. ) ;
#5801=CARTESIAN_POINT ( 'NONE',  ( -74.99999999999997158, 45.00000000000001421, 15.00000000000000000 ) ) ;
#5802=EDGE_CURVE ( 'NONE', #17702, #13670, #18748, .T. ) ;
#5817=VERTEX_POINT ( 'NONE', #2377 ) ;
#5819=ORIENTED_EDGE ( 'NONE', *, *, #3055, .F. ) ;
#5830=CARTESIAN_POINT ( 'NONE',  ( -59.84999999999998721, 32.50000000000001421, 15.00000000000000000 ) ) ;
#5840=ORIENTED_EDGE ( 'NONE', *, *, #1780, .F. ) ;
#5848=EDGE_CURVE ( 'NONE', #2897, #6112, #7643, .T. ) ;
#5879=VERTEX_POINT ( 'NONE', #16290 ) ;
#5885=DIRECTION ( 'NONE',  ( 0.000000000000000000, -0.000000000000000000, 1.000000000000000000 ) ) ;
#5903=DIRECTION ( 'NONE',  ( 0.000000000000000000, 0.000000000000000000, -1.000000000000000000 ) ) ;
#5916=ORIENTED_EDGE ( 'NONE', *, *, #3582, .F. ) ;
#5924=CARTESIAN_POINT ( 'NONE',  ( 62.49999999999998579, 40.00000000000001421, -9.999999999999998224 ) ) ;
#5940=CARTESIAN_POINT ( 'NONE',  ( 32.49999999999998579, 45.00000000000001421, 5.000000000000003553 ) ) ;
#5959=DIRECTION ( 'NONE',  ( 0.000000000000000000, 1.000000000000000000, 0.000000000000000000 ) ) ;
#6010=AXIS2_PLACEMENT_3D ( 'NONE', #3077, #322, #15021 ) ;
#6041=EDGE_CURVE ( 'NONE', #4513, #2192, #2548, .T. ) ;
#6043=CARTESIAN_POINT ( 'NONE',  ( 1.925929944387235853E-31, 15.00000000000001599, 9.999999999999998224 ) ) ;
#6083=VECTOR ( 'NONE', #12695, 1000.000000000000000 ) ;
#6111=ADVANCED_FACE ( 'NONE', ( #16869 ), #6452, .T. ) ;
#6112=VERTEX_POINT ( 'NONE', #7834 ) ;
#6120=CARTESIAN_POINT ( 'NONE',  ( 62.49999999999998579, 5.000000000000018652, -5.000000000000000000 ) ) ;
#6131=ORIENTED_EDGE ( 'NONE', *, *, #17858, .F. ) ;
#6151=ORIENTED_EDGE ( 'NONE', *, *, #9312, .T. ) ;
#6178=CARTESIAN_POINT ( 'NONE',  ( 0.000000000000000000, 20.00000000000001421, -9.999999999999998224 ) ) ;
#6185=VERTEX_POINT ( 'NONE', #5277 ) ;
#6188=ORIENTED_EDGE ( 'NONE', *, *, #17675, .T. ) ;
#6189=LINE ( 'NONE', #12064, #7988 ) ;
#6254=DIRECTION ( 'NONE',  ( 0.000000000000000000, -0.000000000000000000, 1.000000000000000000 ) ) ;
#6276=SHAPE_REPRESENTATION_RELATIONSHIP ( 'NONE' , 'NONE' ,  #659, #8491 ) ;
#6280=SHAPE_DEFINITION_REPRESENTATION ( #14460, #659 ) ;
#6282=VECTOR ( 'NONE', #128, 1000.000000000000000 ) ;
#6290=EDGE_CURVE ( 'NONE', #2561, #17889, #3465, .T. ) ;
#6302=EDGE_CURVE ( 'NONE', #671, #9948, #3914, .T. ) ;
#6314=DIRECTION ( 'NONE',  ( -0.000000000000000000, -0.000000000000000000, 1.000000000000000000 ) ) ;
#6340=DIRECTION ( 'NONE',  ( -0.000000000000000000, -0.000000000000000000, 1.000000000000000000 ) ) ;
#6369=DIRECTION ( 'NONE',  ( -0.000000000000000000, -0.000000000000000000, 1.000000000000000000 ) ) ;
#6397=CARTESIAN_POINT ( 'NONE',  ( 62.49999999999998579, 45.00000000000001421, 15.00000000000000000 ) ) ;
#6414=CARTESIAN_POINT ( 'NONE',  ( 10.00000000000000000, 25.00000000000001776, 15.00000000000000000 ) ) ;
#6422=VERTEX_POINT ( 'NONE', #2932 ) ;
#6425=CIRCLE ( 'NONE', #9244, 2.649999999999985700 ) ;
#6449=CARTESIAN_POINT ( 'NONE',  ( -74.99999999999997158, 32.50000000000001421, 9.999999999999998224 ) ) ;
#6452=PLANE ( 'NONE',  #1594 ) ;
#6471=LINE ( 'NONE', #14010, #8043 ) ;
#6478=DIRECTION ( 'NONE',  ( 0.000000000000000000, -0.000000000000000000, 1.000000000000000000 ) ) ;
#6482=CARTESIAN_POINT ( 'NONE',  ( -74.99999999999997158, 20.00000000000001421, 15.00000000000000000 ) ) ;
#6502=EDGE_CURVE ( 'NONE', #14591, #4513, #8486, .T. ) ;
#6504=ORIENTED_EDGE ( 'NONE', *, *, #4133, .F. ) ;
#6520=CARTESIAN_POINT ( 'NONE',  ( 10.00000000000000000, 20.00000000000001421, 15.00000000000000000 ) ) ;
#6536=EDGE_LOOP ( 'NONE', ( #11374, #8464, #3586, #180 ) ) ;
#6543=CARTESIAN_POINT ( 'NONE',  ( 62.50000000000000000, 32.50000000000001421, 15.00000000000000000 ) ) ;
#6569=DIRECTION ( 'NONE',  ( 0.000000000000000000, -1.000000000000000000, 0.000000000000000000 ) ) ;
#6577=FACE_OUTER_BOUND ( 'NONE', #11225, .T. ) ;
#6581=AXIS2_PLACEMENT_3D ( 'NONE', #16986, #15398, #17076 ) ;
#6591=LINE ( 'NONE', #6397, #9587 ) ;
#6607=VERTEX_POINT ( 'NONE', #3506 ) ;
#6630=VERTEX_POINT ( 'NONE', #15454 ) ;
#6632=DIRECTION ( 'NONE',  ( 0.000000000000000000, 0.000000000000000000, -1.000000000000000000 ) ) ;
#6645=DIRECTION ( 'NONE',  ( -1.000000000000000000, 1.110223024625156935E-15, 0.000000000000000000 ) ) ;
#6651=DIRECTION ( 'NONE',  ( -1.000000000000000000, 0.000000000000000000, 0.000000000000000000 ) ) ;
#6658=EDGE_CURVE ( 'NONE', #6708, #9457, #13797, .T. ) ;
#6696=DIRECTION ( 'NONE',  ( -0.000000000000000000, -0.000000000000000000, 1.000000000000000000 ) ) ;
#6708=VERTEX_POINT ( 'NONE', #946 ) ;
#6733=FACE_OUTER_BOUND ( 'NONE', #10350, .T. ) ;
#6785=AXIS2_PLACEMENT_3D ( 'NONE', #4102, #5663, #4393 ) ;
#6802=FACE_OUTER_BOUND ( 'NONE', #7792, .T. ) ;
#6839=CIRCLE ( 'NONE', #17820, 2.649999999999988365 ) ;
#6840=DIRECTION ( 'NONE',  ( 0.000000000000000000, 0.000000000000000000, -1.000000000000000000 ) ) ;
#6858=CARTESIAN_POINT ( 'NONE',  ( -9.999999999999994671, 20.00000000000001421, 15.00000000000000000 ) ) ;
#6871=FACE_OUTER_BOUND ( 'NONE', #19005, .T. ) ;
#6878=DIRECTION ( 'NONE',  ( -0.000000000000000000, -0.000000000000000000, -1.000000000000000000 ) ) ;
#6893=ORIENTED_EDGE ( 'NONE', *, *, #1614, .T. ) ;
#6897=ORIENTED_EDGE ( 'NONE', *, *, #8320, .F. ) ;
#6922=ORIENTED_EDGE ( 'NONE', *, *, #14905, .T. ) ;
#6925=VERTEX_POINT ( 'NONE', #5940 ) ;
#6946=ORIENTED_EDGE ( 'NONE', *, *, #8565, .T. ) ;
#6978=CARTESIAN_POINT ( 'NONE',  ( 0.000000000000000000, 0.000000000000000000, -9.999999999999998224 ) ) ;
#6981=DIRECTION ( 'NONE',  ( 0.000000000000000000, 0.000000000000000000, -1.000000000000000000 ) ) ;
#6986=CARTESIAN_POINT ( 'NONE',  ( 62.49999999999998579, 45.00000000000001421, 9.999999999999998224 ) ) ;
#7017=VERTEX_POINT ( 'NONE', #13573 ) ;
#7032=DIRECTION ( 'NONE',  ( 0.000000000000000000, 0.000000000000000000, -1.000000000000000000 ) ) ;
#7039=EDGE_CURVE ( 'NONE', #4201, #8542, #17275, .T. ) ;
#7049=ORIENTED_EDGE ( 'NONE', *, *, #3582, .T. ) ;
#7070=CARTESIAN_POINT ( 'NONE',  ( -9.999999999999996447, 25.00000000000001776, 15.00000000000000000 ) ) ;
#7075=VERTEX_POINT ( 'NONE', #4851 ) ;
#7090=VECTOR ( 'NONE', #6314, 1000.000000000000000 ) ;
#7100=CLOSED_SHELL ( 'NONE', ( #12631, #11831, #18693, #15165, #9269, #16229, #17676, #2633, #10725, #68, #16303, #11112, #8303, #2982, #16106, #8285, #4003, #8699, #4247, #16011, #19312, #1618, #18572, #16493, #1721, #3774, #13649, #6111, #903, #14042, #3659, #7400, #2230, #1488, #1613, #7128, #12747, #11270 ) ) ;
#7104=CYLINDRICAL_SURFACE ( 'NONE', #11825, 9.999999999999998224 ) ;
#7116=EDGE_LOOP ( 'NONE', ( #2642, #18730, #4086, #8468 ) ) ;
#7124=ORIENTED_EDGE ( 'NONE', *, *, #16523, .F. ) ;
#7127=LINE ( 'NONE', #14104, #16932 ) ;
#7128=ADVANCED_FACE ( 'NONE', ( #3959 ), #14236, .F. ) ;
#7129=VERTEX_POINT ( 'NONE', #6986 ) ;
#7131=ORIENTED_EDGE ( 'NONE', *, *, #5452, .F. ) ;
#7147=DIRECTION ( 'NONE',  ( -0.000000000000000000, -0.000000000000000000, 1.000000000000000000 ) ) ;
#7155=DIRECTION ( 'NONE',  ( 1.000000000000000000, 0.000000000000000000, 0.000000000000000000 ) ) ;
#7183=DIRECTION ( 'NONE',  ( -1.000000000000000000, 0.000000000000000000, 0.000000000000000000 ) ) ;
#7195=ORIENTED_EDGE ( 'NONE', *, *, #17675, .F. ) ;
#7200=DIRECTION ( 'NONE',  ( 0.000000000000000000, 0.000000000000000000, -1.000000000000000000 ) ) ;
#7203=CARTESIAN_POINT ( 'NONE',  ( 62.49999999999998579, 20.00000000000001421, -15.00000000000000000 ) ) ;
#7210=DIRECTION ( 'NONE',  ( -1.000000000000000000, 0.000000000000000000, -0.000000000000000000 ) ) ;
#7214=ORIENTED_EDGE ( 'NONE', *, *, #17441, .T. ) ;
#7224=ORIENTED_EDGE ( 'NONE', *, *, #19127, .F. ) ;
#7238=EDGE_CURVE ( 'NONE', #15661, #4513, #2103, .T. ) ;
#7247=DIRECTION ( 'NONE',  ( -1.000000000000000000, 0.000000000000000000, 0.000000000000000000 ) ) ;
#7275=DIRECTION ( 'NONE',  ( 1.000000000000000000, 0.000000000000000000, 0.000000000000000000 ) ) ;
#7286=CARTESIAN_POINT ( 'NONE',  ( 62.49999999999998579, 45.00000000000001421, 5.000000000000000000 ) ) ;
#7287=ORIENTED_EDGE ( 'NONE', *, *, #15036, .F. ) ;
#7332=VECTOR ( 'NONE', #17195, 1000.000000000000000 ) ;
#7345=UNCERTAINTY_MEASURE_WITH_UNIT (LENGTH_MEASURE( 1.000000000000000082E-05 ), #10583, 'distance_accuracy_value', 'NONE');
#7359=EDGE_CURVE ( 'NONE', #12330, #6630, #4358, .T. ) ;
#7387=ORIENTED_EDGE ( 'NONE', *, *, #11676, .T. ) ;
#7388=CIRCLE ( 'NONE', #18366, 2.649999999999988365 ) ;
#7400=ADVANCED_FACE ( 'NONE', ( #1623 ), #11995, .F. ) ;
#7405=CARTESIAN_POINT ( 'NONE',  ( 0.000000000000000000, 0.000000000000000000, -15.00000000000000000 ) ) ;
#7417=EDGE_CURVE ( 'NONE', #11786, #17308, #18198, .T. ) ;
#7426=CYLINDRICAL_SURFACE ( 'NONE', #846, 12.49999999999999645 ) ;
#7458=EDGE_CURVE ( 'NONE', #14591, #3708, #7776, .T. ) ;
#7481=ORIENTED_EDGE ( 'NONE', *, *, #15267, .F. ) ;
#7492=CARTESIAN_POINT ( 'NONE',  ( -9.999999999999994671, 20.00000000000001421, 15.00000000000000000 ) ) ;
#7514=EDGE_LOOP ( 'NONE', ( #1239, #3441, #10246, #18615 ) ) ;
#7534=VECTOR ( 'NONE', #2356, 1000.000000000000000 ) ;
#7551=CIRCLE ( 'NONE', #10981, 12.49999999999999645 ) ;
#7557=ORIENTED_EDGE ( 'NONE', *, *, #3307, .F. ) ;
#7562=LINE ( 'NONE', #10876, #5018 ) ;
#7563=VECTOR ( 'NONE', #13041, 1000.000000000000000 ) ;
#7574=VERTEX_POINT ( 'NONE', #12374 ) ;
#7584=ORIENTED_EDGE ( 'NONE', *, *, #4477, .T. ) ;
#7617=EDGE_CURVE ( 'NONE', #11648, #10528, #6591, .T. ) ;
#7626=DIRECTION ( 'NONE',  ( 1.000000000000000000, -0.000000000000000000, 0.000000000000000000 ) ) ;
#7643=LINE ( 'NONE', #6178, #1315 ) ;
#7652=CARTESIAN_POINT ( 'NONE',  ( 62.49999999999998579, 45.00000000000001421, 0.000000000000000000 ) ) ;
#7654=CARTESIAN_POINT ( 'NONE',  ( 62.50000000000000000, 32.50000000000001421, 9.999999999999998224 ) ) ;
#7673=ORIENTED_EDGE ( 'NONE', *, *, #10566, .F. ) ;
#7677=ORIENTED_EDGE ( 'NONE', *, *, #11907, .F. ) ;
#7678=DIRECTION ( 'NONE',  ( -1.000000000000000000, 0.000000000000000000, 1.224646799147353207E-16 ) ) ;
#7694=ORIENTED_EDGE ( 'NONE', *, *, #14779, .T. ) ;
#7700=DIRECTION ( 'NONE',  ( -0.000000000000000000, -0.000000000000000000, 1.000000000000000000 ) ) ;
#7706=LINE ( 'NONE', #13685, #18261 ) ;
#7738=DIRECTION ( 'NONE',  ( 0.000000000000000000, 0.000000000000000000, 1.000000000000000000 ) ) ;
#7740=CARTESIAN_POINT ( 'NONE',  ( 62.49999999999998579, 45.00000000000001421, 0.000000000000000000 ) ) ;
#7744=EDGE_LOOP ( 'NONE', ( #10973, #6946, #14302, #11154 ) ) ;
#7771=( GEOMETRIC_REPRESENTATION_CONTEXT ( 3 ) GLOBAL_UNCERTAINTY_ASSIGNED_CONTEXT ( ( #10279 ) ) GLOBAL_UNIT_ASSIGNED_CONTEXT ( ( #17868, #4136, #7930 ) ) REPRESENTATION_CONTEXT ( 'NONE', 'WORKASPACE' ) );
#7776=LINE ( 'NONE', #13474, #7090 ) ;
#7778=DIRECTION ( 'NONE',  ( -0.000000000000000000, -0.000000000000000000, 1.000000000000000000 ) ) ;
#7784=DIRECTION ( 'NONE',  ( 0.000000000000000000, 0.000000000000000000, -1.000000000000000000 ) ) ;
#7789=ORIENTED_EDGE ( 'NONE', *, *, #7039, .T. ) ;
#7791=LINE ( 'NONE', #3294, #10732 ) ;
#7792=EDGE_LOOP ( 'NONE', ( #18822, #13695, #7287, #18409 ) ) ;
#7826=VECTOR ( 'NONE', #4939, 1000.000000000000000 ) ;
#7829=CARTESIAN_POINT ( 'NONE',  ( -74.99999999999997158, 20.00000000000001421, 15.00000000000000000 ) ) ;
#7834=CARTESIAN_POINT ( 'NONE',  ( 62.50000000000000000, 20.00000000000001421, -9.999999999999998224 ) ) ;
#7844=( NAMED_UNIT ( * ) SI_UNIT ( $, .STERADIAN. ) SOLID_ANGLE_UNIT ( ) );
#7847=ORIENTED_EDGE ( 'NONE', *, *, #16374, .T. ) ;
#7857=DIRECTION ( 'NONE',  ( -1.000000000000000000, 0.000000000000000000, -0.000000000000000000 ) ) ;
#7868=AXIS2_PLACEMENT_3D ( 'NONE', #3763, #6696, #5418 ) ;
#7873=VERTEX_POINT ( 'NONE', #4608 ) ;
#7891=EDGE_LOOP ( 'NONE', ( #9935, #2214, #3323, #4886 ) ) ;
#7892=CARTESIAN_POINT ( 'NONE',  ( 62.49999999999998579, 32.50000000000001421, 9.999999999999998224 ) ) ;
#7905=AXIS2_PLACEMENT_3D ( 'NONE', #15136, #11803, #15230 ) ;
#7925=DIRECTION ( 'NONE',  ( -1.000000000000000000, 0.000000000000000000, 0.000000000000000000 ) ) ;
#7930=( NAMED_UNIT ( * ) SI_UNIT ( $, .STERADIAN. ) SOLID_ANGLE_UNIT ( ) );
#7957=FACE_OUTER_BOUND ( 'NONE', #17157, .T. ) ;
#7972=CARTESIAN_POINT ( 'NONE',  ( 10.00000000000000000, 25.00000000000001776, -15.00000000000000000 ) ) ;
#7978=CARTESIAN_POINT ( 'NONE',  ( -2.649999999999988365, 15.00000000000001599, 15.00000000000000000 ) ) ;
#7984=CARTESIAN_POINT ( 'NONE',  ( 62.49999999999998579, 45.00000000000001421, -5.000000000000000000 ) ) ;
#7988=VECTOR ( 'NONE', #15112, 1000.000000000000000 ) ;
#7991=CARTESIAN_POINT ( 'NONE',  ( -9.999999999999998224, 15.00000000000001776, 15.00000000000000000 ) ) ;
#8008=AXIS2_PLACEMENT_3D ( 'NONE', #19025, #3715, #11539 ) ;
#8012=DIRECTION ( 'NONE',  ( 0.000000000000000000, 1.000000000000000000, 0.000000000000000000 ) ) ;
#8034=CARTESIAN_POINT ( 'NONE',  ( 10.00000000000000000, 25.00000000000001776, 15.00000000000000000 ) ) ;
#8043=VECTOR ( 'NONE', #10984, 1000.000000000000000 ) ;
#8046=AXIS2_PLACEMENT_3D ( 'NONE', #14518, #1103, #17192 ) ;
#8076=( GEOMETRIC_REPRESENTATION_CONTEXT ( 3 ) GLOBAL_UNCERTAINTY_ASSIGNED_CONTEXT ( ( #16763 ) ) GLOBAL_UNIT_ASSIGNED_CONTEXT ( ( #18357, #3343, #7844 ) ) REPRESENTATION_CONTEXT ( 'NONE', 'WORKASPACE' ) );
#8091=CARTESIAN_POINT ( 'NONE',  ( -62.49999999999997158, 32.50000000000001421, 9.999999999999998224 ) ) ;
#8097=FACE_BOUND ( 'NONE', #11984, .T. ) ;
#8100=ORIENTED_EDGE ( 'NONE', *, *, #6502, .F. ) ;
#8104=CYLINDRICAL_SURFACE ( 'NONE', #364, 12.49999999999999645 ) ;
#8123=DIRECTION ( 'NONE',  ( -0.000000000000000000, 0.000000000000000000, -1.000000000000000000 ) ) ;
#8128=VECTOR ( 'NONE', #1682, 1000.000000000000000 ) ;
#8203=VECTOR ( 'NONE', #14203, 1000.000000000000000 ) ;
#8218=CARTESIAN_POINT ( 'NONE',  ( 1.925929944387235853E-31, 15.00000000000001599, -15.00000000000000000 ) ) ;
#8219=ORIENTED_EDGE ( 'NONE', *, *, #7417, .F. ) ;
#8275=LINE ( 'NONE', #9461, #6083 ) ;
#8285=ADVANCED_FACE ( 'NONE', ( #8889 ), #4195, .F. ) ;
#8303=ADVANCED_FACE ( 'NONE', ( #15966 ), #7426, .T. ) ;
#8307=CARTESIAN_POINT ( 'NONE',  ( -74.99999999999997158, 20.00000000000001421, 15.00000000000000000 ) ) ;
#8320=EDGE_CURVE ( 'NONE', #7574, #4179, #1351, .T. ) ;
#8348=DIRECTION ( 'NONE',  ( -1.000000000000000000, 0.000000000000000000, -0.000000000000000000 ) ) ;
#8354=FACE_OUTER_BOUND ( 'NONE', #985, .T. ) ;
#8405=AXIS2_PLACEMENT_3D ( 'NONE', #9850, #17235, #9949 ) ;
#8413=CARTESIAN_POINT ( 'NONE',  ( -62.49999999999997158, 32.50000000000001421, 15.00000000000000178 ) ) ;
#8422=DIRECTION ( 'NONE',  ( 0.000000000000000000, 0.000000000000000000, -1.000000000000000000 ) ) ;
#8464=ORIENTED_EDGE ( 'NONE', *, *, #4133, .T. ) ;
#8468=ORIENTED_EDGE ( 'NONE', *, *, #5310, .F. ) ;
#8480=CIRCLE ( 'NONE', #2859, 2.649999999999987477 ) ;
#8486=CIRCLE ( 'NONE', #14425, 12.49999999999999645 ) ;
#8491=ADVANCED_BREP_SHAPE_REPRESENTATION ( '', ( #14815, #10359 ), #7771 ) ;
#8498=ORIENTED_EDGE ( 'NONE', *, *, #16881, .T. ) ;
#8504=CIRCLE ( 'NONE', #6010, 12.49999999999999645 ) ;
#8511=DIRECTION ( 'NONE',  ( -0.000000000000000000, -0.000000000000000000, 1.000000000000000000 ) ) ;
#8523=LINE ( 'NONE', #14492, #13099 ) ;
#8542=VERTEX_POINT ( 'NONE', #17128 ) ;
#8544=DIRECTION ( 'NONE',  ( -0.000000000000000000, -0.000000000000000000, 1.000000000000000000 ) ) ;
#8565=EDGE_CURVE ( 'NONE', #6708, #6185, #12499, .T. ) ;
#8566=ORIENTED_EDGE ( 'NONE', *, *, #3062, .T. ) ;
#8571=DIRECTION ( 'NONE',  ( -1.000000000000000000, 0.000000000000000000, 0.000000000000000000 ) ) ;
#8615=CARTESIAN_POINT ( 'NONE',  ( 2.649999999999988365, 15.00000000000001599, -9.999999999999998224 ) ) ;
#8684=DIRECTION ( 'NONE',  ( -0.000000000000000000, 1.000000000000000000, -0.000000000000000000 ) ) ;
#8688=VECTOR ( 'NONE', #5292, 1000.000000000000000 ) ;
#8699=ADVANCED_FACE ( 'NONE', ( #11415 ), #7104, .T. ) ;
#8729=VERTEX_POINT ( 'NONE', #7203 ) ;
#8741=CARTESIAN_POINT ( 'NONE',  ( 62.49999999999998579, 40.00000000000001421, 5.000000000000000000 ) ) ;
#8755=ORIENTED_EDGE ( 'NONE', *, *, #7238, .F. ) ;
#8817=ORIENTED_EDGE ( 'NONE', *, *, #15749, .T. ) ;
#8824=CARTESIAN_POINT ( 'NONE',  ( 62.49999999999998579, 45.00000000000001421, 15.00000000000000000 ) ) ;
#8834=DIRECTION ( 'NONE',  ( 0.000000000000000000, 0.000000000000000000, 1.000000000000000000 ) ) ;
#8839=DIRECTION ( 'NONE',  ( 1.000000000000000000, 0.000000000000000000, 0.000000000000000000 ) ) ;
#8840=CARTESIAN_POINT ( 'NONE',  ( -2.649999999999988365, 15.00000000000001599, 15.00000000000000000 ) ) ;
#8863=EDGE_LOOP ( 'NONE', ( #19279, #17987, #2133, #19186 ) ) ;
#8879=EDGE_LOOP ( 'NONE', ( #4070, #12391, #12227, #6893 ) ) ;
#8882=VECTOR ( 'NONE', #7778, 1000.000000000000000 ) ;
#8883=ORIENTED_EDGE ( 'NONE', *, *, #7359, .T. ) ;
#8889=FACE_OUTER_BOUND ( 'NONE', #3907, .T. ) ;
#8895=ORIENTED_EDGE ( 'NONE', *, *, #4237, .T. ) ;
#8982=LINE ( 'NONE', #9079, #15101 ) ;
#9004=ORIENTED_EDGE ( 'NONE', *, *, #14050, .F. ) ;
#9021=EDGE_CURVE ( 'NONE', #6185, #5879, #12681, .T. ) ;
#9027=CARTESIAN_POINT ( 'NONE',  ( 62.50000000000000000, 32.50000000000001421, 15.00000000000000000 ) ) ;
#9031=CARTESIAN_POINT ( 'NONE',  ( 32.49999999999998579, 5.000000000000018652, 5.000000000000003553 ) ) ;
#9052=EDGE_LOOP ( 'NONE', ( #16319, #15565, #16298, #17823 ) ) ;
#9070=VERTEX_POINT ( 'NONE', #12461 ) ;
#9079=CARTESIAN_POINT ( 'NONE',  ( -62.49999999999997158, 45.00000000000001421, -9.999999999999998224 ) ) ;
#9099=CARTESIAN_POINT ( 'NONE',  ( 62.49999999999998579, 32.50000000000001421, 15.00000000000000000 ) ) ;
#9105=ORIENTED_EDGE ( 'NONE', *, *, #10704, .T. ) ;
#9125=ORIENTED_EDGE ( 'NONE', *, *, #2957, .T. ) ;
#9155=CARTESIAN_POINT ( 'NONE',  ( -9.999999999999998224, 15.00000000000001776, 15.00000000000000000 ) ) ;
#9215=CARTESIAN_POINT ( 'NONE',  ( 0.000000000000000000, 40.00000000000001421, -9.999999999999998224 ) ) ;
#9244=AXIS2_PLACEMENT_3D ( 'NONE', #1485, #6369, #3164 ) ;
#9264=EDGE_CURVE ( 'NONE', #7873, #10516, #6425, .T. ) ;
#9269=ADVANCED_FACE ( 'NONE', ( #11969 ), #16495, .T. ) ;
#9273=AXIS2_PLACEMENT_3D ( 'NONE', #6120, #12187, #7678 ) ;
#9285=EDGE_CURVE ( 'NONE', #2433, #10922, #10688, .T. ) ;
#9301=EDGE_LOOP ( 'NONE', ( #15902, #4501, #6151, #1116 ) ) ;
#9312=EDGE_CURVE ( 'NONE', #2433, #9835, #6189, .T. ) ;
#9371=CARTESIAN_POINT ( 'NONE',  ( -9.999999999999994671, 20.00000000000001421, 9.999999999999998224 ) ) ;
#9393=EDGE_CURVE ( 'NONE', #17702, #3410, #10874, .T. ) ;
#9399=ORIENTED_EDGE ( 'NONE', *, *, #3648, .F. ) ;
#9457=VERTEX_POINT ( 'NONE', #5284 ) ;
#9461=CARTESIAN_POINT ( 'NONE',  ( 62.49999999999998579, 45.00000000000001421, 5.000000000000000000 ) ) ;
#9479=ORIENTED_EDGE ( 'NONE', *, *, #18031, .T. ) ;
#9486=DIRECTION ( 'NONE',  ( 1.000000000000000000, 0.000000000000000000, 0.000000000000000000 ) ) ;
#9490=VERTEX_POINT ( 'NONE', #18646 ) ;
#9495=CARTESIAN_POINT ( 'NONE',  ( -9.999999999999996447, 25.00000000000001776, 15.00000000000000000 ) ) ;
#9519=VECTOR ( 'NONE', #1184, 1000.000000000000000 ) ;
#9530=DIRECTION ( 'NONE',  ( -0.000000000000000000, 0.000000000000000000, -1.000000000000000000 ) ) ;
#9587=VECTOR ( 'NONE', #11091, 1000.000000000000000 ) ;
#9596=FACE_BOUND ( 'NONE', #17040, .T. ) ;
#9616=CARTESIAN_POINT ( 'NONE',  ( -74.99999999999997158, 20.00000000000001421, -15.00000000000000000 ) ) ;
#9637=DIRECTION ( 'NONE',  ( -0.000000000000000000, -0.000000000000000000, 1.000000000000000000 ) ) ;
#9639=DIRECTION ( 'NONE',  ( -1.000000000000000000, 0.000000000000000000, 0.000000000000000000 ) ) ;
#9656=LINE ( 'NONE', #15105, #8128 ) ;
#9667=ORIENTED_EDGE ( 'NONE', *, *, #16660, .F. ) ;
#9776=ORIENTED_EDGE ( 'NONE', *, *, #4974, .F. ) ;
#9777=CARTESIAN_POINT ( 'NONE',  ( -74.99999999999997158, 20.00000000000001421, 15.00000000000000000 ) ) ;
#9797=CARTESIAN_POINT ( 'NONE',  ( 32.49999999999998579, 40.00000000000001421, -4.999999999999996447 ) ) ;
#9810=VECTOR ( 'NONE', #9530, 1000.000000000000000 ) ;
#9815=CYLINDRICAL_SURFACE ( 'NONE', #4532, 9.999999999999998224 ) ;
#9834=CARTESIAN_POINT ( 'NONE',  ( 9.999999999999994671, 20.00000000000001421, 9.999999999999998224 ) ) ;
#9835=VERTEX_POINT ( 'NONE', #15090 ) ;
#9850=CARTESIAN_POINT ( 'NONE',  ( 62.50000000000000000, 32.50000000000001421, -15.00000000000000000 ) ) ;
#9853=VECTOR ( 'NONE', #4497, 1000.000000000000000 ) ;
#9862=AXIS2_PLACEMENT_3D ( 'NONE', #7652, #4628, #16782 ) ;
#9891=CARTESIAN_POINT ( 'NONE',  ( -74.99999999999997158, 20.00000000000001421, -15.00000000000000000 ) ) ;
#9928=ORIENTED_EDGE ( 'NONE', *, *, #12262, .T. ) ;
#9935=ORIENTED_EDGE ( 'NONE', *, *, #2217, .T. ) ;
#9948=VERTEX_POINT ( 'NONE', #3705 ) ;
#9949=DIRECTION ( 'NONE',  ( -1.000000000000000000, 0.000000000000000000, 0.000000000000000000 ) ) ;
#9958=ORIENTED_EDGE ( 'NONE', *, *, #12641, .T. ) ;
#9964=DIRECTION ( 'NONE',  ( 0.000000000000000000, 1.000000000000000000, 0.000000000000000000 ) ) ;
#9985=LINE ( 'NONE', #14793, #14091 ) ;
#10075=PRODUCT ( 'idle-roller mover', 'idle-roller mover', '', ( #16981 ) ) ;
#10077=ORIENTED_EDGE ( 'NONE', *, *, #10935, .F. ) ;
#10152=ORIENTED_EDGE ( 'NONE', *, *, #16523, .T. ) ;
#10166=AXIS2_PLACEMENT_3D ( 'NONE', #13594, #6340, #12117 ) ;
#10179=DIRECTION ( 'NONE',  ( 1.000000000000000000, -0.000000000000000000, 0.000000000000000000 ) ) ;
#10200=PLANE ( 'NONE',  #12337 ) ;
#10208=CARTESIAN_POINT ( 'NONE',  ( 9.999999999999994671, 20.00000000000001421, 15.00000000000000000 ) ) ;
#10232=DIRECTION ( 'NONE',  ( -0.000000000000000000, -0.000000000000000000, -1.000000000000000000 ) ) ;
#10246=ORIENTED_EDGE ( 'NONE', *, *, #2723, .F. ) ;
#10275=AXIS2_PLACEMENT_3D ( 'NONE', #8413, #7147, #14393 ) ;
#10279=UNCERTAINTY_MEASURE_WITH_UNIT (LENGTH_MEASURE( 1.000000000000000082E-05 ), #17868, 'distance_accuracy_value', 'NONE');
#10334=AXIS2_PLACEMENT_3D ( 'NONE', #17117, #11110, #12591 ) ;
#10350=EDGE_LOOP ( 'NONE', ( #5178, #19382, #8755, #2022 ) ) ;
#10359=AXIS2_PLACEMENT_3D ( 'NONE', #2871, #8834, #16191 ) ;
#10459=PLANE ( 'NONE',  #19394 ) ;
#10470=ORIENTED_EDGE ( 'NONE', *, *, #1970, .F. ) ;
#10506=ORIENTED_EDGE ( 'NONE', *, *, #10704, .F. ) ;
#10509=AXIS2_PLACEMENT_3D ( 'NONE', #10961, #7738, #9486 ) ;
#10512=CARTESIAN_POINT ( 'NONE',  ( -62.49999999999997158, 20.00000000000001421, -9.999999999999998224 ) ) ;
#10516=VERTEX_POINT ( 'NONE', #16926 ) ;
#10528=VERTEX_POINT ( 'NONE', #1825 ) ;
#10566=EDGE_CURVE ( 'NONE', #14864, #12519, #5332, .T. ) ;
#10583=( LENGTH_UNIT ( ) NAMED_UNIT ( * ) SI_UNIT ( .MILLI., .METRE. ) );
#10584=EDGE_CURVE ( 'NONE', #17741, #7129, #1900, .T. ) ;
#10586=EDGE_LOOP ( 'NONE', ( #6131, #2981, #11427, #10077, #8883, #5093, #11000, #10152, #17365, #7694, #18915, #15669 ) ) ;
#10611=AXIS2_PLACEMENT_3D ( 'NONE', #16420, #227, #15126 ) ;
#10612=CIRCLE ( 'NONE', #2814, 2.649999999999988365 ) ;
#10673=AXIS2_PLACEMENT_3D ( 'NONE', #6543, #14183, #6645 ) ;
#10677=AXIS2_PLACEMENT_3D ( 'NONE', #2646, #8511, #14481 ) ;
#10688=LINE ( 'NONE', #9215, #804 ) ;
#10693=AXIS2_PLACEMENT_3D ( 'NONE', #15452, #4693, #13876 ) ;
#10704=EDGE_CURVE ( 'NONE', #8542, #4201, #16008, .T. ) ;
#10725=ADVANCED_FACE ( 'NONE', ( #6802 ), #5234, .T. ) ;
#10732=VECTOR ( 'NONE', #2112, 1000.000000000000000 ) ;
#10763=ORIENTED_EDGE ( 'NONE', *, *, #10566, .T. ) ;
#10779=ORIENTED_EDGE ( 'NONE', *, *, #14905, .F. ) ;
#10784=CARTESIAN_POINT ( 'NONE',  ( -59.84999999999998721, 32.50000000000001421, 15.00000000000000178 ) ) ;
#10785=DIRECTION ( 'NONE',  ( 0.000000000000000000, 0.000000000000000000, 1.000000000000000000 ) ) ;
#10814=VERTEX_POINT ( 'NONE', #10512 ) ;
#10817=CIRCLE ( 'NONE', #10509, 9.999999999999998224 ) ;
#10822=CARTESIAN_POINT ( 'NONE',  ( 62.50000000000000000, 20.00000000000001421, 15.00000000000000000 ) ) ;
#10856=PRODUCT_DEFINITION_CONTEXT ( 'detailed design', #11024, 'design' ) ;
#10874=LINE ( 'NONE', #9495, #17726 ) ;
#10876=CARTESIAN_POINT ( 'NONE',  ( 0.000000000000000000, 40.00000000000001421, 9.999999999999998224 ) ) ;
#10883=FACE_OUTER_BOUND ( 'NONE', #12912, .T. ) ;
#10909=DIRECTION ( 'NONE',  ( -1.000000000000000000, 0.000000000000000000, 0.000000000000000000 ) ) ;
#10922=VERTEX_POINT ( 'NONE', #5924 ) ;
#10935=EDGE_CURVE ( 'NONE', #12330, #7075, #16222, .T. ) ;
#10937=DIRECTION ( 'NONE',  ( -1.000000000000000000, 0.000000000000000000, 0.000000000000000000 ) ) ;
#10956=VECTOR ( 'NONE', #2725, 1000.000000000000000 ) ;
#10957=EDGE_CURVE ( 'NONE', #10814, #2113, #7551, .T. ) ;
#10961=CARTESIAN_POINT ( 'NONE',  ( 1.925929944387235853E-31, 15.00000000000001599, 15.00000000000000000 ) ) ;
#10973=ORIENTED_EDGE ( 'NONE', *, *, #6658, .F. ) ;
#10974=DIRECTION ( 'NONE',  ( 0.000000000000000000, -1.000000000000000000, 0.000000000000000000 ) ) ;
#10980=CARTESIAN_POINT ( 'NONE',  ( 62.49999999999998579, 40.00000000000001421, -5.000000000000000000 ) ) ;
#10981=AXIS2_PLACEMENT_3D ( 'NONE', #15035, #1617, #13562 ) ;
#10984=DIRECTION ( 'NONE',  ( -0.000000000000000000, 1.000000000000000000, -0.000000000000000000 ) ) ;
#11000=ORIENTED_EDGE ( 'NONE', *, *, #7458, .T. ) ;
#11015=CARTESIAN_POINT ( 'NONE',  ( 62.49999999999998579, 32.50000000000001421, -9.999999999999998224 ) ) ;
#11017=DIRECTION ( 'NONE',  ( -0.000000000000000000, 1.000000000000000000, -0.000000000000000000 ) ) ;
#11024=APPLICATION_CONTEXT ( 'automotive_design' ) ;
#11033=CARTESIAN_POINT ( 'NONE',  ( 32.49999999999998579, 45.00000000000001421, -4.999999999999996447 ) ) ;
#11057=EDGE_CURVE ( 'NONE', #178, #10922, #12422, .T. ) ;
#11070=CARTESIAN_POINT ( 'NONE',  ( -9.999999999999994671, 20.00000000000001421, -15.00000000000000000 ) ) ;
#11072=CIRCLE ( 'NONE', #17990, 12.49999999999999645 ) ;
#11074=EDGE_CURVE ( 'NONE', #11811, #2802, #18432, .T. ) ;
#11087=LINE ( 'NONE', #9616, #933 ) ;
#11091=DIRECTION ( 'NONE',  ( -0.000000000000000000, 0.000000000000000000, -1.000000000000000000 ) ) ;
#11092=LINE ( 'NONE', #13849, #2967 ) ;
#11102=DIRECTION ( 'NONE',  ( -0.000000000000000000, -0.000000000000000000, 1.000000000000000000 ) ) ;
#11110=DIRECTION ( 'NONE',  ( 0.000000000000000000, 0.000000000000000000, -1.000000000000000000 ) ) ;
#11112=ADVANCED_FACE ( 'NONE', ( #6733 ), #8104, .T. ) ;
#11139=CARTESIAN_POINT ( 'NONE',  ( -62.49999999999997158, 32.50000000000001421, 15.00000000000000000 ) ) ;
#11154=ORIENTED_EDGE ( 'NONE', *, *, #16881, .F. ) ;
#11225=EDGE_LOOP ( 'NONE', ( #9399, #16642, #2457, #10506 ) ) ;
#11227=ORIENTED_EDGE ( 'NONE', *, *, #2137, .F. ) ;
#11228=CARTESIAN_POINT ( 'NONE',  ( 0.000000000000000000, 0.000000000000000000, 9.999999999999998224 ) ) ;
#11270=ADVANCED_FACE ( 'NONE', ( #18919 ), #16064, .F. ) ;
#11312=DIRECTION ( 'NONE',  ( -1.000000000000000000, 0.000000000000000000, 0.000000000000000000 ) ) ;
#11323=DIRECTION ( 'NONE',  ( -0.000000000000000000, -0.000000000000000000, -1.000000000000000000 ) ) ;
#11341=ORIENTED_EDGE ( 'NONE', *, *, #118, .T. ) ;
#11344=CIRCLE ( 'NONE', #2913, 12.49999999999999645 ) ;
#11356=DIRECTION ( 'NONE',  ( -0.000000000000000000, -0.000000000000000000, 1.000000000000000000 ) ) ;
#11365=EDGE_CURVE ( 'NONE', #2561, #14864, #13679, .T. ) ;
#11374=ORIENTED_EDGE ( 'NONE', *, *, #5802, .T. ) ;
#11403=EDGE_CURVE ( 'NONE', #273, #9070, #4438, .T. ) ;
#11407=ORIENTED_EDGE ( 'NONE', *, *, #12800, .F. ) ;
#11415=FACE_OUTER_BOUND ( 'NONE', #7744, .T. ) ;
#11427=ORIENTED_EDGE ( 'NONE', *, *, #5122, .T. ) ;
#11438=ORIENTED_EDGE ( 'NONE', *, *, #8565, .F. ) ;
#11458=PLANE ( 'NONE',  #15174 ) ;
#11472=AXIS2_PLACEMENT_3D ( 'NONE', #9027, #14818, #7275 ) ;
#11483=CARTESIAN_POINT ( 'NONE',  ( -62.49999999999997158, 32.50000000000001421, -15.00000000000000000 ) ) ;
#11492=ORIENTED_EDGE ( 'NONE', *, *, #13598, .T. ) ;
#11508=DIRECTION ( 'NONE',  ( 0.000000000000000000, 0.000000000000000000, -1.000000000000000000 ) ) ;
#11512=COLOUR_RGB ( '',0.8941176470588234615, 0.8941176470588234615, 0.8941176470588234615 ) ;
#11521=CIRCLE ( 'NONE', #12161, 12.49999999999999645 ) ;
#11527=EDGE_LOOP ( 'NONE', ( #17462, #7214, #7049, #2240 ) ) ;
#11531=DIRECTION ( 'NONE',  ( 0.000000000000000000, 0.000000000000000000, -1.000000000000000000 ) ) ;
#11539=DIRECTION ( 'NONE',  ( -1.000000000000000000, 0.000000000000000000, 1.224646799147353207E-16 ) ) ;
#11558=FACE_OUTER_BOUND ( 'NONE', #18062, .T. ) ;
#11574=LINE ( 'NONE', #5801, #17863 ) ;
#11595=VECTOR ( 'NONE', #13889, 1000.000000000000000 ) ;
#11624=AXIS2_PLACEMENT_3D ( 'NONE', #17704, #1125, #13079 ) ;
#11648=VERTEX_POINT ( 'NONE', #7984 ) ;
#11676=EDGE_CURVE ( 'NONE', #3708, #15661, #680, .T. ) ;
#11692=CARTESIAN_POINT ( 'NONE',  ( -74.99999999999997158, 20.00000000000001421, 15.00000000000000000 ) ) ;
#11696=DIRECTION ( 'NONE',  ( 1.000000000000000000, 0.000000000000000000, 0.000000000000000000 ) ) ;
#11710=ORIENTED_EDGE ( 'NONE', *, *, #9393, .T. ) ;
#11725=CARTESIAN_POINT ( 'NONE',  ( 62.50000000000000000, 20.00000000000001421, 15.00000000000000000 ) ) ;
#11763=FACE_OUTER_BOUND ( 'NONE', #6536, .T. ) ;
#11771=DIRECTION ( 'NONE',  ( 1.000000000000000000, 0.000000000000000000, 0.000000000000000000 ) ) ;
#11782=ORIENTED_EDGE ( 'NONE', *, *, #9021, .F. ) ;
#11784=ORIENTED_EDGE ( 'NONE', *, *, #2825, .F. ) ;
#11786=VERTEX_POINT ( 'NONE', #14250 ) ;
#11803=DIRECTION ( 'NONE',  ( 0.000000000000000000, 1.000000000000000000, 0.000000000000000000 ) ) ;
#11811=VERTEX_POINT ( 'NONE', #9834 ) ;
#11825=AXIS2_PLACEMENT_3D ( 'NONE', #13087, #10232, #19095 ) ;
#11831=ADVANCED_FACE ( 'NONE', ( #15935 ), #5732, .F. ) ;
#11883=ORIENTED_EDGE ( 'NONE', *, *, #4897, .F. ) ;
#11885=CYLINDRICAL_SURFACE ( 'NONE', #10611, 12.49999999999999645 ) ;
#11888=ORIENTED_EDGE ( 'NONE', *, *, #18278, .T. ) ;
#11907=EDGE_CURVE ( 'NONE', #10814, #248, #4753, .T. ) ;
#11921=VECTOR ( 'NONE', #3516, 1000.000000000000000 ) ;
#11969=FACE_OUTER_BOUND ( 'NONE', #8863, .T. ) ;
#11984=EDGE_LOOP ( 'NONE', ( #3328, #2143 ) ) ;
#11995=PLANE ( 'NONE',  #9273 ) ;
#12003=FACE_BOUND ( 'NONE', #232, .T. ) ;
#12006=CARTESIAN_POINT ( 'NONE',  ( 62.49999999999998579, 5.000000000000018652, 5.000000000000000000 ) ) ;
#12064=CARTESIAN_POINT ( 'NONE',  ( -62.49999999999997158, 40.00000000000001421, 0.000000000000000000 ) ) ;
#12117=DIRECTION ( 'NONE',  ( 1.000000000000000000, 0.000000000000000000, 0.000000000000000000 ) ) ;
#12132=DIRECTION ( 'NONE',  ( -0.000000000000000000, -0.000000000000000000, 1.000000000000000000 ) ) ;
#12133=ORIENTED_EDGE ( 'NONE', *, *, #5452, .T. ) ;
#12161=AXIS2_PLACEMENT_3D ( 'NONE', #9099, #12132, #7247 ) ;
#12184=CARTESIAN_POINT ( 'NONE',  ( 75.00000000000000000, 32.50000000000001421, 9.999999999999998224 ) ) ;
#12187=DIRECTION ( 'NONE',  ( -1.224646799147353207E-16, 0.000000000000000000, -1.000000000000000000 ) ) ;
#12193=VECTOR ( 'NONE', #5312, 1000.000000000000000 ) ;
#12203=DIRECTION ( 'NONE',  ( -0.000000000000000000, -0.000000000000000000, 1.000000000000000000 ) ) ;
#12214=DIRECTION ( 'NONE',  ( 1.000000000000000000, 0.000000000000000000, 0.000000000000000000 ) ) ;
#12227=ORIENTED_EDGE ( 'NONE', *, *, #11057, .T. ) ;
#12262=EDGE_CURVE ( 'NONE', #15125, #3771, #2121, .T. ) ;
#12299=CARTESIAN_POINT ( 'NONE',  ( 1.925929944387235853E-31, 15.00000000000001599, -9.999999999999998224 ) ) ;
#12330=VERTEX_POINT ( 'NONE', #13153 ) ;
#12337=AXIS2_PLACEMENT_3D ( 'NONE', #6978, #1203, #8348 ) ;
#12344=FILL_AREA_STYLE ('',( #304 ) ) ;
#12351=AXIS2_PLACEMENT_3D ( 'NONE', #104, #17857, #14895 ) ;
#12374=CARTESIAN_POINT ( 'NONE',  ( 32.49999999999998579, 40.00000000000001421, 5.000000000000002665 ) ) ;
#12391=ORIENTED_EDGE ( 'NONE', *, *, #540, .F. ) ;
#12422=LINE ( 'NONE', #12621, #11921 ) ;
#12451=FACE_BOUND ( 'NONE', #2895, .T. ) ;
#12461=CARTESIAN_POINT ( 'NONE',  ( -65.14999999999996305, 32.50000000000001421, 15.00000000000000178 ) ) ;
#12499=LINE ( 'NONE', #7991, #13073 ) ;
#12519=VERTEX_POINT ( 'NONE', #16079 ) ;
#12540=EDGE_LOOP ( 'NONE', ( #1724, #4163, #8100, #1298, #3799, #11492, #13613, #13308, #5269, #12565, #14455, #6504 ) ) ;
#12562=CARTESIAN_POINT ( 'NONE',  ( -62.49999999999997158, 32.50000000000001421, 15.00000000000000000 ) ) ;
#12565=ORIENTED_EDGE ( 'NONE', *, *, #4680, .F. ) ;
#12567=DIRECTION ( 'NONE',  ( 0.000000000000000000, 0.000000000000000000, 1.000000000000000000 ) ) ;
#12591=DIRECTION ( 'NONE',  ( -1.000000000000000000, 0.000000000000000000, 0.000000000000000000 ) ) ;
#12614=CARTESIAN_POINT ( 'NONE',  ( 1.925929944387235853E-31, 15.00000000000001599, 15.00000000000000000 ) ) ;
#12621=CARTESIAN_POINT ( 'NONE',  ( 62.49999999999998579, 40.00000000000001421, 0.000000000000000000 ) ) ;
#12631=ADVANCED_FACE ( 'NONE', ( #980 ), #5773, .F. ) ;
#12635=ORIENTED_EDGE ( 'NONE', *, *, #18280, .F. ) ;
#12641=EDGE_CURVE ( 'NONE', #178, #4179, #4013, .T. ) ;
#12643=ORIENTED_EDGE ( 'NONE', *, *, #12641, .F. ) ;
#12645=CIRCLE ( 'NONE', #5129, 12.49999999999999645 ) ;
#12652=CYLINDRICAL_SURFACE ( 'NONE', #14623, 2.649999999999988365 ) ;
#12664=DIRECTION ( 'NONE',  ( 0.000000000000000000, 1.000000000000000000, 0.000000000000000000 ) ) ;
#12681=CIRCLE ( 'NONE', #18656, 9.999999999999998224 ) ;
#12695=DIRECTION ( 'NONE',  ( -1.000000000000000000, 0.000000000000000000, 1.224646799147353207E-16 ) ) ;
#12729=EDGE_LOOP ( 'NONE', ( #2914, #7584 ) ) ;
#12743=CARTESIAN_POINT ( 'NONE',  ( 62.50000000000000000, 20.00000000000001421, 9.999999999999998224 ) ) ;
#12747=ADVANCED_FACE ( 'NONE', ( #6577 ), #17087, .F. ) ;
#12749=CARTESIAN_POINT ( 'NONE',  ( 10.00000000000000000, 0.000000000000000000, -9.999999999999998224 ) ) ;
#12758=AXIS2_PLACEMENT_3D ( 'NONE', #5196, #3355, #7857 ) ;
#12761=DIRECTION ( 'NONE',  ( 1.000000000000000000, 0.000000000000000000, 0.000000000000000000 ) ) ;
#12780=ORIENTED_EDGE ( 'NONE', *, *, #15267, .T. ) ;
#12788=DIRECTION ( 'NONE',  ( -0.000000000000000000, 0.000000000000000000, -1.000000000000000000 ) ) ;
#12800=EDGE_CURVE ( 'NONE', #16565, #164, #3939, .T. ) ;
#12815=EDGE_LOOP ( 'NONE', ( #4989, #7224, #5366, #4555 ) ) ;
#12823=VECTOR ( 'NONE', #8684, 1000.000000000000000 ) ;
#12847=AXIS2_PLACEMENT_3D ( 'NONE', #7892, #3675, #9639 ) ;
#12869=CARTESIAN_POINT ( 'NONE',  ( -62.49999999999997158, 45.00000000000001421, 15.00000000000000000 ) ) ;
#12870=EDGE_CURVE ( 'NONE', #5817, #9490, #2587, .T. ) ;
#12904=LINE ( 'NONE', #14363, #10956 ) ;
#12911=ORIENTED_EDGE ( 'NONE', *, *, #14173, .F. ) ;
#12912=EDGE_LOOP ( 'NONE', ( #2830, #11710, #3437, #17134, #17636, #6188, #18709, #7124, #7387, #2922 ) ) ;
#12975=ORIENTED_EDGE ( 'NONE', *, *, #11907, .T. ) ;
#13018=FACE_OUTER_BOUND ( 'NONE', #5101, .T. ) ;
#13031=ORIENTED_EDGE ( 'NONE', *, *, #16374, .F. ) ;
#13041=DIRECTION ( 'NONE',  ( -0.000000000000000000, 0.000000000000000000, -1.000000000000000000 ) ) ;
#13073=VECTOR ( 'NONE', #11323, 1000.000000000000000 ) ;
#13076=VERTEX_POINT ( 'NONE', #3158 ) ;
#13079=DIRECTION ( 'NONE',  ( -1.000000000000000000, 0.000000000000000000, 0.000000000000000000 ) ) ;
#13087=CARTESIAN_POINT ( 'NONE',  ( 1.925929944387235853E-31, 15.00000000000001599, 15.00000000000000000 ) ) ;
#13099=VECTOR ( 'NONE', #2459, 1000.000000000000000 ) ;
#13129=AXIS2_PLACEMENT_3D ( 'NONE', #3673, #9637, #15635 ) ;
#13135=DIRECTION ( 'NONE',  ( -0.000000000000000000, 1.000000000000000000, -0.000000000000000000 ) ) ;
#13153=CARTESIAN_POINT ( 'NONE',  ( -62.49999999999997158, 45.00000000000001421, -15.00000000000000000 ) ) ;
#13160=AXIS2_PLACEMENT_3D ( 'NONE', #18209, #11102, #14040 ) ;
#13195=LINE ( 'NONE', #12006, #12823 ) ;
#13204=EDGE_LOOP ( 'NONE', ( #15858, #19105, #5370, #7847 ) ) ;
#13218=DIRECTION ( 'NONE',  ( 0.000000000000000000, 1.000000000000000000, 0.000000000000000000 ) ) ;
#13264=CARTESIAN_POINT ( 'NONE',  ( -62.49999999999997158, 45.00000000000001421, 9.999999999999998224 ) ) ;
#13272=DIRECTION ( 'NONE',  ( 0.000000000000000000, 0.000000000000000000, -1.000000000000000000 ) ) ;
#13282=VECTOR ( 'NONE', #6569, 1000.000000000000000 ) ;
#13293=CIRCLE ( 'NONE', #12351, 2.649999999999985700 ) ;
#13297=CARTESIAN_POINT ( 'NONE',  ( -62.49999999999997158, 32.50000000000001421, 15.00000000000000178 ) ) ;
#13308=ORIENTED_EDGE ( 'NONE', *, *, #16599, .F. ) ;
#13324=CARTESIAN_POINT ( 'NONE',  ( 75.00000000000000000, 32.50000000000001421, 15.00000000000000000 ) ) ;
#13364=DIRECTION ( 'NONE',  ( 0.000000000000000000, -0.000000000000000000, 1.000000000000000000 ) ) ;
#13389=EDGE_CURVE ( 'NONE', #6630, #14591, #8523, .T. ) ;
#13447=CARTESIAN_POINT ( 'NONE',  ( -74.99999999999997158, 32.50000000000001421, 15.00000000000000000 ) ) ;
#13470=ORIENTED_EDGE ( 'NONE', *, *, #6290, .T. ) ;
#13474=CARTESIAN_POINT ( 'NONE',  ( -62.49999999999997158, 45.00000000000001421, 15.00000000000000000 ) ) ;
#13562=DIRECTION ( 'NONE',  ( -1.000000000000000000, 0.000000000000000000, 0.000000000000000000 ) ) ;
#13573=CARTESIAN_POINT ( 'NONE',  ( 62.49999999999998579, 45.00000000000001421, 15.00000000000000000 ) ) ;
#13594=CARTESIAN_POINT ( 'NONE',  ( 1.925929944387235853E-31, 15.00000000000001599, -15.00000000000000000 ) ) ;
#13598=EDGE_CURVE ( 'NONE', #16565, #7129, #15085, .T. ) ;
#13613=ORIENTED_EDGE ( 'NONE', *, *, #10584, .F. ) ;
#13614=LINE ( 'NONE', #14990, #16629 ) ;
#13626=LINE ( 'NONE', #18158, #19124 ) ;
#13649=ADVANCED_FACE ( 'NONE', ( #1457 ), #10459, .F. ) ;
#13654=EDGE_LOOP ( 'NONE', ( #7789, #9105 ) ) ;
#13659=DIRECTION ( 'NONE',  ( -0.000000000000000000, 0.000000000000000000, -1.000000000000000000 ) ) ;
#13670=VERTEX_POINT ( 'NONE', #9371 ) ;
#13677=VECTOR ( 'NONE', #15164, 1000.000000000000000 ) ;
#13679=LINE ( 'NONE', #4487, #5052 ) ;
#13685=CARTESIAN_POINT ( 'NONE',  ( 62.49999999999998579, 5.000000000000018652, -5.000000000000000000 ) ) ;
#13695=ORIENTED_EDGE ( 'NONE', *, *, #14355, .T. ) ;
#13734=DIRECTION ( 'NONE',  ( 1.000000000000000000, 0.000000000000000000, 0.000000000000000000 ) ) ;
#13797=CIRCLE ( 'NONE', #18835, 9.999999999999998224 ) ;
#13831=FACE_OUTER_BOUND ( 'NONE', #13884, .T. ) ;
#13839=CARTESIAN_POINT ( 'NONE',  ( -74.99999999999997158, 45.00000000000001421, 15.00000000000000000 ) ) ;
#13849=CARTESIAN_POINT ( 'NONE',  ( -59.84999999999998721, 32.50000000000001421, 15.00000000000000000 ) ) ;
#13876=DIRECTION ( 'NONE',  ( -1.000000000000000000, 0.000000000000000000, 0.000000000000000000 ) ) ;
#13884=EDGE_LOOP ( 'NONE', ( #4280, #15461, #1955, #4649 ) ) ;
#13889=DIRECTION ( 'NONE',  ( 1.000000000000000000, -0.000000000000000000, 0.000000000000000000 ) ) ;
#13896=CARTESIAN_POINT ( 'NONE',  ( -74.99999999999997158, 32.50000000000001421, -9.999999999999998224 ) ) ;
#13903=( NAMED_UNIT ( * ) SI_UNIT ( $, .STERADIAN. ) SOLID_ANGLE_UNIT ( ) );
#13911=CARTESIAN_POINT ( 'NONE',  ( -62.49999999999997158, 20.00000000000001421, -15.00000000000000000 ) ) ;
#13927=PLANE ( 'NONE',  #1567 ) ;
#13929=EDGE_CURVE ( 'NONE', #6422, #8729, #19087, .T. ) ;
#13939=LINE ( 'NONE', #3565, #9810 ) ;
#14010=CARTESIAN_POINT ( 'NONE',  ( 62.49999999999998579, 0.000000000000000000, -9.999999999999998224 ) ) ;
#14012=STYLED_ITEM ( 'NONE', ( #4623 ), #8491 ) ;
#14018=CIRCLE ( 'NONE', #10275, 2.649999999999985700 ) ;
#14019=VECTOR ( 'NONE', #13218, 1000.000000000000000 ) ;
#14040=DIRECTION ( 'NONE',  ( 1.000000000000000000, 0.000000000000000000, 0.000000000000000000 ) ) ;
#14042=ADVANCED_FACE ( 'NONE', ( #8097, #5257, #2134 ), #14074, .T. ) ;
#14050=EDGE_CURVE ( 'NONE', #18826, #62, #6839, .T. ) ;
#14066=AXIS2_PLACEMENT_3D ( 'NONE', #7654, #211, #18361 ) ;
#14074=PLANE ( 'NONE',  #4673 ) ;
#14078=ORIENTED_EDGE ( 'NONE', *, *, #4507, .F. ) ;
#14091=VECTOR ( 'NONE', #10179, 1000.000000000000000 ) ;
#14104=CARTESIAN_POINT ( 'NONE',  ( 10.00000000000000000, 15.00000000000001776, 15.00000000000000000 ) ) ;
#14112=CARTESIAN_POINT ( 'NONE',  ( 10.00000000000000000, 25.00000000000001776, 15.00000000000000000 ) ) ;
#14143=ORIENTED_EDGE ( 'NONE', *, *, #4680, .T. ) ;
#14164=DIRECTION ( 'NONE',  ( -0.000000000000000000, -0.000000000000000000, 1.000000000000000000 ) ) ;
#14173=EDGE_CURVE ( 'NONE', #164, #19088, #13195, .T. ) ;
#14183=DIRECTION ( 'NONE',  ( -0.000000000000000000, -0.000000000000000000, 1.000000000000000000 ) ) ;
#14203=DIRECTION ( 'NONE',  ( -0.000000000000000000, -0.000000000000000000, 1.000000000000000000 ) ) ;
#14215=EDGE_CURVE ( 'NONE', #12519, #14864, #10612, .T. ) ;
#14236=CYLINDRICAL_SURFACE ( 'NONE', #7868, 2.649999999999988365 ) ;
#14250=CARTESIAN_POINT ( 'NONE',  ( -9.999999999999994671, 20.00000000000001421, -9.999999999999998224 ) ) ;
#14251=ORIENTED_EDGE ( 'NONE', *, *, #1780, .T. ) ;
#14284=PLANE ( 'NONE',  #8008 ) ;
#14302=ORIENTED_EDGE ( 'NONE', *, *, #9021, .T. ) ;
#14320=DIRECTION ( 'NONE',  ( 0.000000000000000000, -0.000000000000000000, 1.000000000000000000 ) ) ;
#14330=CARTESIAN_POINT ( 'NONE',  ( 75.00000000000000000, 32.50000000000001421, -9.999999999999998224 ) ) ;
#14332=CARTESIAN_POINT ( 'NONE',  ( 62.49999999999998579, 32.50000000000001421, 15.00000000000000000 ) ) ;
#14355=EDGE_CURVE ( 'NONE', #10528, #5263, #308, .T. ) ;
#14363=CARTESIAN_POINT ( 'NONE',  ( -74.99999999999997158, 40.00000000000001421, 5.000000000000018652 ) ) ;
#14393=DIRECTION ( 'NONE',  ( 1.000000000000000000, 0.000000000000000000, 0.000000000000000000 ) ) ;
#14415=CARTESIAN_POINT ( 'NONE',  ( 10.00000000000000000, 15.00000000000001776, 15.00000000000000000 ) ) ;
#14425=AXIS2_PLACEMENT_3D ( 'NONE', #8091, #16846, #10937 ) ;
#14455=ORIENTED_EDGE ( 'NONE', *, *, #17138, .F. ) ;
#14460=PRODUCT_DEFINITION_SHAPE ( 'NONE', 'NONE',  #1359 ) ;
#14481=DIRECTION ( 'NONE',  ( 1.000000000000000000, 0.000000000000000000, 0.000000000000000000 ) ) ;
#14487=CARTESIAN_POINT ( 'NONE',  ( -62.49999999999997158, 20.00000000000001421, 9.999999999999998224 ) ) ;
#14492=CARTESIAN_POINT ( 'NONE',  ( -62.49999999999997158, 45.00000000000001421, 15.00000000000000000 ) ) ;
#14518=CARTESIAN_POINT ( 'NONE',  ( -62.49999999999997158, 32.50000000000001421, 9.999999999999998224 ) ) ;
#14541=DIRECTION ( 'NONE',  ( -0.000000000000000000, -0.000000000000000000, 1.000000000000000000 ) ) ;
#14574=DIRECTION ( 'NONE',  ( -1.000000000000000000, 0.000000000000000000, 0.000000000000000000 ) ) ;
#14591=VERTEX_POINT ( 'NONE', #13264 ) ;
#14623=AXIS2_PLACEMENT_3D ( 'NONE', #17081, #16991, #13734 ) ;
#14625=ORIENTED_EDGE ( 'NONE', *, *, #15134, .F. ) ;
#14630=FACE_OUTER_BOUND ( 'NONE', #3896, .T. ) ;
#14718=CARTESIAN_POINT ( 'NONE',  ( 2.649999999999988365, 15.00000000000001599, 9.999999999999998224 ) ) ;
#14731=VECTOR ( 'NONE', #3090, 1000.000000000000000 ) ;
#14734=ORIENTED_EDGE ( 'NONE', *, *, #15610, .F. ) ;
#14737=ORIENTED_EDGE ( 'NONE', *, *, #14215, .T. ) ;
#14739=ORIENTED_EDGE ( 'NONE', *, *, #5310, .T. ) ;
#14773=LINE ( 'NONE', #1452, #1381 ) ;
#14779=EDGE_CURVE ( 'NONE', #7129, #19088, #16876, .T. ) ;
#14793=CARTESIAN_POINT ( 'NONE',  ( 0.000000000000000000, 20.00000000000001421, 9.999999999999998224 ) ) ;
#14815=MANIFOLD_SOLID_BREP ( 'M5 Clearance Hole1', #7100 ) ;
#14818=DIRECTION ( 'NONE',  ( 0.000000000000000000, -0.000000000000000000, 1.000000000000000000 ) ) ;
#14851=EDGE_CURVE ( 'NONE', #62, #4248, #981, .T. ) ;
#14864=VERTEX_POINT ( 'NONE', #8615 ) ;
#14895=DIRECTION ( 'NONE',  ( 1.000000000000000000, 0.000000000000000000, 0.000000000000000000 ) ) ;
#14905=EDGE_CURVE ( 'NONE', #9070, #273, #14018, .T. ) ;
#14932=PLANE ( 'NONE',  #418 ) ;
#14946=VECTOR ( 'NONE', #2079, 1000.000000000000000 ) ;
#14981=LINE ( 'NONE', #2620, #1518 ) ;
#14990=CARTESIAN_POINT ( 'NONE',  ( -9.999999999999996447, 25.00000000000001776, -15.00000000000000000 ) ) ;
#15004=( NAMED_UNIT ( * ) PLANE_ANGLE_UNIT ( ) SI_UNIT ( $, .RADIAN. ) );
#15021=DIRECTION ( 'NONE',  ( -1.000000000000000000, 0.000000000000000000, 0.000000000000000000 ) ) ;
#15035=CARTESIAN_POINT ( 'NONE',  ( -62.49999999999997158, 32.50000000000001421, -9.999999999999998224 ) ) ;
#15036=EDGE_CURVE ( 'NONE', #6422, #5263, #14981, .T. ) ;
#15064=AXIS2_PLACEMENT_3D ( 'NONE', #9777, #8012, #474 ) ;
#15067=DIRECTION ( 'NONE',  ( 1.000000000000000000, 0.000000000000000000, 0.000000000000000000 ) ) ;
#15072=FACE_OUTER_BOUND ( 'NONE', #7514, .T. ) ;
#15085=LINE ( 'NONE', #2937, #14019 ) ;
#15090=CARTESIAN_POINT ( 'NONE',  ( -62.49999999999997158, 40.00000000000001421, 9.999999999999998224 ) ) ;
#15101=VECTOR ( 'NONE', #5959, 1000.000000000000000 ) ;
#15105=CARTESIAN_POINT ( 'NONE',  ( -65.14999999999996305, 32.50000000000001421, 15.00000000000000000 ) ) ;
#15112=DIRECTION ( 'NONE',  ( -0.000000000000000000, 0.000000000000000000, 1.000000000000000000 ) ) ;
#15125=VERTEX_POINT ( 'NONE', #16564 ) ;
#15126=DIRECTION ( 'NONE',  ( 1.000000000000000000, 0.000000000000000000, 0.000000000000000000 ) ) ;
#15134=EDGE_CURVE ( 'NONE', #6607, #7017, #11521, .T. ) ;
#15136=CARTESIAN_POINT ( 'NONE',  ( -74.99999999999997158, 40.00000000000001421, 15.00000000000000000 ) ) ;
#15151=CARTESIAN_POINT ( 'NONE',  ( -74.99999999999997158, 32.50000000000001421, 15.00000000000000000 ) ) ;
#15152=ORIENTED_EDGE ( 'NONE', *, *, #5802, .F. ) ;
#15164=DIRECTION ( 'NONE',  ( 0.000000000000000000, 1.000000000000000000, 0.000000000000000000 ) ) ;
#15165=ADVANCED_FACE ( 'NONE', ( #18528 ), #2042, .F. ) ;
#15174=AXIS2_PLACEMENT_3D ( 'NONE', #15793, #992, #5487 ) ;
#15200=EDGE_LOOP ( 'NONE', ( #3527, #9004 ) ) ;
#15216=CARTESIAN_POINT ( 'NONE',  ( -74.99999999999997158, 40.00000000000001421, -4.999999999999984013 ) ) ;
#15230=DIRECTION ( 'NONE',  ( 0.000000000000000000, -0.000000000000000000, 1.000000000000000000 ) ) ;
#15254=LINE ( 'NONE', #16654, #13677 ) ;
#15267=EDGE_CURVE ( 'NONE', #11811, #671, #3322, .T. ) ;
#15297=EDGE_LOOP ( 'NONE', ( #16381, #9479, #7673, #2933 ) ) ;
#15306=FACE_OUTER_BOUND ( 'NONE', #18638, .T. ) ;
#15343=AXIS2_PLACEMENT_3D ( 'NONE', #7405, #16532, #7210 ) ;
#15398=DIRECTION ( 'NONE',  ( -0.000000000000000000, -0.000000000000000000, 1.000000000000000000 ) ) ;
#15410=DIRECTION ( 'NONE',  ( 0.000000000000000000, 1.000000000000000000, 0.000000000000000000 ) ) ;
#15452=CARTESIAN_POINT ( 'NONE',  ( -62.49999999999997158, 32.50000000000001421, -9.999999999999998224 ) ) ;
#15454=CARTESIAN_POINT ( 'NONE',  ( -62.49999999999997158, 45.00000000000001421, -9.999999999999998224 ) ) ;
#15461=ORIENTED_EDGE ( 'NONE', *, *, #6290, .F. ) ;
#15465=DIRECTION ( 'NONE',  ( 0.000000000000000000, 0.000000000000000000, -1.000000000000000000 ) ) ;
#15487=VECTOR ( 'NONE', #9964, 1000.000000000000000 ) ;
#15540=ORIENTED_EDGE ( 'NONE', *, *, #10935, .T. ) ;
#15542=DIRECTION ( 'NONE',  ( 1.000000000000000000, -0.000000000000000000, 0.000000000000000000 ) ) ;
#15551=ORIENTED_EDGE ( 'NONE', *, *, #17858, .T. ) ;
#15561=ORIENTED_EDGE ( 'NONE', *, *, #9285, .T. ) ;
#15564=AXIS2_PLACEMENT_3D ( 'NONE', #15835, #14541, #11696 ) ;
#15565=ORIENTED_EDGE ( 'NONE', *, *, #3648, .T. ) ;
#15610=EDGE_CURVE ( 'NONE', #7574, #6925, #7791, .T. ) ;
#15614=VECTOR ( 'NONE', #6254, 1000.000000000000000 ) ;
#15635=DIRECTION ( 'NONE',  ( -1.000000000000000000, 0.000000000000000000, 0.000000000000000000 ) ) ;
#15651=EDGE_CURVE ( 'NONE', #18826, #13076, #18215, .T. ) ;
#15661=VERTEX_POINT ( 'NONE', #15151 ) ;
#15669=ORIENTED_EDGE ( 'NONE', *, *, #4897, .T. ) ;
#15724=CARTESIAN_POINT ( 'NONE',  ( -74.99999999999997158, 32.50000000000001421, 15.00000000000000000 ) ) ;
#15736=EDGE_CURVE ( 'NONE', #5817, #671, #16923, .T. ) ;
#15749=EDGE_CURVE ( 'NONE', #2802, #9948, #2016, .T. ) ;
#15770=CARTESIAN_POINT ( 'NONE',  ( 0.000000000000000000, 20.00000000000001421, 9.999999999999998224 ) ) ;
#15783=DIRECTION ( 'NONE',  ( 1.000000000000000000, 0.000000000000000000, 0.000000000000000000 ) ) ;
#15793=CARTESIAN_POINT ( 'NONE',  ( -74.99999999999997158, 20.00000000000001421, 15.00000000000000000 ) ) ;
#15804=VECTOR ( 'NONE', #291, 1000.000000000000000 ) ;
#15814=CARTESIAN_POINT ( 'NONE',  ( 1.925929944387235853E-31, 15.00000000000001599, 15.00000000000000000 ) ) ;
#15835=CARTESIAN_POINT ( 'NONE',  ( -62.49999999999997158, 32.50000000000001421, 15.00000000000000000 ) ) ;
#15836=ORIENTED_EDGE ( 'NONE', *, *, #11057, .F. ) ;
#15858=ORIENTED_EDGE ( 'NONE', *, *, #15651, .F. ) ;
#15885=EDGE_CURVE ( 'NONE', #15661, #1247, #2812, .T. ) ;
#15890=CARTESIAN_POINT ( 'NONE',  ( -59.84999999999998721, 32.50000000000001421, -9.999999999999998224 ) ) ;
#15902=ORIENTED_EDGE ( 'NONE', *, *, #13389, .F. ) ;
#15935=FACE_OUTER_BOUND ( 'NONE', #9052, .T. ) ;
#15966=FACE_OUTER_BOUND ( 'NONE', #7116, .T. ) ;
#16007=DIRECTION ( 'NONE',  ( -0.000000000000000000, 0.000000000000000000, -1.000000000000000000 ) ) ;
#16008=CIRCLE ( 'NONE', #350, 2.649999999999985700 ) ;
#16011=ADVANCED_FACE ( 'NONE', ( #4162 ), #14932, .F. ) ;
#16064=CYLINDRICAL_SURFACE ( 'NONE', #10677, 2.649999999999985700 ) ;
#16066=LINE ( 'NONE', #11725, #8203 ) ;
#16079=CARTESIAN_POINT ( 'NONE',  ( -2.649999999999988365, 15.00000000000001599, -9.999999999999998224 ) ) ;
#16089=LINE ( 'NONE', #12749, #8688 ) ;
#16106=ADVANCED_FACE ( 'NONE', ( #14630 ), #11885, .T. ) ;
#16110=FACE_BOUND ( 'NONE', #13654, .T. ) ;
#16154=EDGE_LOOP ( 'NONE', ( #18884, #16367, #11782, #5608, #19016, #12133, #14739, #15540, #4999, #533 ) ) ;
#16191=DIRECTION ( 'NONE',  ( 1.000000000000000000, 0.000000000000000000, 0.000000000000000000 ) ) ;
#16222=LINE ( 'NONE', #17701, #14731 ) ;
#16228=DIRECTION ( 'NONE',  ( -1.000000000000000000, 0.000000000000000000, 0.000000000000000000 ) ) ;
#16229=ADVANCED_FACE ( 'NONE', ( #7957 ), #13927, .F. ) ;
#16248=ORIENTED_EDGE ( 'NONE', *, *, #18280, .T. ) ;
#16290=CARTESIAN_POINT ( 'NONE',  ( 10.00000000000000000, 15.00000000000001776, -15.00000000000000000 ) ) ;
#16292=AXIS2_PLACEMENT_3D ( 'NONE', #16301, #8544, #1487 ) ;
#16298=ORIENTED_EDGE ( 'NONE', *, *, #7039, .F. ) ;
#16301=CARTESIAN_POINT ( 'NONE',  ( 1.925929944387235853E-31, 15.00000000000001599, 15.00000000000000178 ) ) ;
#16303=ADVANCED_FACE ( 'NONE', ( #6871 ), #711, .T. ) ;
#16319=ORIENTED_EDGE ( 'NONE', *, *, #4477, .F. ) ;
#16324=ORIENTED_EDGE ( 'NONE', *, *, #1614, .F. ) ;
#16334=AXIS2_PLACEMENT_3D ( 'NONE', #13297, #16448, #15067 ) ;
#16367=ORIENTED_EDGE ( 'NONE', *, *, #18699, .F. ) ;
#16374=EDGE_CURVE ( 'NONE', #4248, #13076, #3140, .T. ) ;
#16381=ORIENTED_EDGE ( 'NONE', *, *, #534, .F. ) ;
#16420=CARTESIAN_POINT ( 'NONE',  ( -62.49999999999997158, 32.50000000000001421, 15.00000000000000000 ) ) ;
#16448=DIRECTION ( 'NONE',  ( -0.000000000000000000, -0.000000000000000000, 1.000000000000000000 ) ) ;
#16465=CARTESIAN_POINT ( 'NONE',  ( -62.49999999999997158, 45.00000000000001421, 0.000000000000000000 ) ) ;
#16481=DIRECTION ( 'NONE',  ( -0.000000000000000000, 0.000000000000000000, -1.000000000000000000 ) ) ;
#16493=ADVANCED_FACE ( 'NONE', ( #11763 ), #5501, .F. ) ;
#16495=PLANE ( 'NONE',  #9862 ) ;
#16508=LINE ( 'NONE', #10208, #6282 ) ;
#16523=EDGE_CURVE ( 'NONE', #3708, #7017, #11574, .T. ) ;
#16532=DIRECTION ( 'NONE',  ( 0.000000000000000000, 0.000000000000000000, -1.000000000000000000 ) ) ;
#16535=DIRECTION ( 'NONE',  ( -1.000000000000000000, 0.000000000000000000, 0.000000000000000000 ) ) ;
#16558=MECHANICAL_DESIGN_GEOMETRIC_PRESENTATION_REPRESENTATION('',(#574),#8076);
#16564=CARTESIAN_POINT ( 'NONE',  ( -59.84999999999998721, 32.50000000000001421, 9.999999999999998224 ) ) ;
#16565=VERTEX_POINT ( 'NONE', #3256 ) ;
#16595=LINE ( 'NONE', #13447, #2437 ) ;
#16596=AXIS2_PLACEMENT_3D ( 'NONE', #3554, #18577, #12761 ) ;
#16599=EDGE_CURVE ( 'NONE', #2802, #17741, #4388, .T. ) ;
#16608=PLANE ( 'NONE',  #18517 ) ;
#16629=VECTOR ( 'NONE', #16674, 1000.000000000000000 ) ;
#16634=FACE_BOUND ( 'NONE', #12729, .T. ) ;
#16642=ORIENTED_EDGE ( 'NONE', *, *, #9264, .F. ) ;
#16654=CARTESIAN_POINT ( 'NONE',  ( -62.49999999999997158, 45.00000000000001421, 9.999999999999998224 ) ) ;
#16660=EDGE_CURVE ( 'NONE', #9835, #16565, #7562, .T. ) ;
#16663=ORIENTED_EDGE ( 'NONE', *, *, #17138, .T. ) ;
#16674=DIRECTION ( 'NONE',  ( 0.000000000000000000, -1.000000000000000000, 0.000000000000000000 ) ) ;
#16695=CARTESIAN_POINT ( 'NONE',  ( -9.999999999999996447, 0.000000000000000000, 9.999999999999998224 ) ) ;
#16696=PLANE ( 'NONE',  #17466 ) ;
#16763=UNCERTAINTY_MEASURE_WITH_UNIT (LENGTH_MEASURE( 1.000000000000000082E-05 ), #18357, 'distance_accuracy_value', 'NONE');
#16782=DIRECTION ( 'NONE',  ( -0.000000000000000000, 0.000000000000000000, -1.000000000000000000 ) ) ;
#16846=DIRECTION ( 'NONE',  ( -0.000000000000000000, -0.000000000000000000, 1.000000000000000000 ) ) ;
#16848=AXIS2_PLACEMENT_3D ( 'NONE', #8034, #18365, #3452 ) ;
#16869=FACE_OUTER_BOUND ( 'NONE', #8879, .T. ) ;
#16871=ORIENTED_EDGE ( 'NONE', *, *, #15736, .F. ) ;
#16876=LINE ( 'NONE', #17068, #4993 ) ;
#16881=EDGE_CURVE ( 'NONE', #9457, #5879, #7127, .T. ) ;
#16904=VECTOR ( 'NONE', #12203, 1000.000000000000000 ) ;
#16923=LINE ( 'NONE', #6414, #599 ) ;
#16926=CARTESIAN_POINT ( 'NONE',  ( -65.14999999999996305, 32.50000000000001421, -15.00000000000000000 ) ) ;
#16932=VECTOR ( 'NONE', #2272, 1000.000000000000000 ) ;
#16945=EDGE_LOOP ( 'NONE', ( #1674, #835, #2311, #7195 ) ) ;
#16969=CARTESIAN_POINT ( 'NONE',  ( -62.49999999999997158, 32.50000000000001421, 9.999999999999998224 ) ) ;
#16981=PRODUCT_CONTEXT ( 'NONE', #18288, 'mechanical' ) ;
#16986=CARTESIAN_POINT ( 'NONE',  ( 1.925929944387235853E-31, 15.00000000000001599, 9.999999999999998224 ) ) ;
#16991=DIRECTION ( 'NONE',  ( -0.000000000000000000, -0.000000000000000000, 1.000000000000000000 ) ) ;
#17000=CARTESIAN_POINT ( 'NONE',  ( 1.925929944387235853E-31, 15.00000000000001599, -15.00000000000000000 ) ) ;
#17022=DIRECTION ( 'NONE',  ( -1.000000000000000000, 0.000000000000000000, 0.000000000000000000 ) ) ;
#17040=EDGE_LOOP ( 'NONE', ( #18090, #10779 ) ) ;
#17068=CARTESIAN_POINT ( 'NONE',  ( 62.49999999999998579, 45.00000000000001421, 15.00000000000000000 ) ) ;
#17073=EDGE_LOOP ( 'NONE', ( #851, #5456, #11883, #14734 ) ) ;
#17076=DIRECTION ( 'NONE',  ( -1.000000000000000000, 0.000000000000000000, 0.000000000000000000 ) ) ;
#17081=CARTESIAN_POINT ( 'NONE',  ( 1.925929944387235853E-31, 15.00000000000001599, 15.00000000000000000 ) ) ;
#17087=CYLINDRICAL_SURFACE ( 'NONE', #3700, 2.649999999999985700 ) ;
#17100=DIRECTION ( 'NONE',  ( -0.000000000000000000, -0.000000000000000000, 1.000000000000000000 ) ) ;
#17117=CARTESIAN_POINT ( 'NONE',  ( 1.925929944387235853E-31, 15.00000000000001599, -9.999999999999998224 ) ) ;
#17122=ORIENTED_EDGE ( 'NONE', *, *, #18452, .F. ) ;
#17128=CARTESIAN_POINT ( 'NONE',  ( -65.14999999999996305, 32.50000000000001421, -9.999999999999998224 ) ) ;
#17134=ORIENTED_EDGE ( 'NONE', *, *, #15736, .T. ) ;
#17138=EDGE_CURVE ( 'NONE', #1462, #9490, #642, .T. ) ;
#17157=EDGE_LOOP ( 'NONE', ( #1705, #12975, #8895, #8219 ) ) ;
#17192=DIRECTION ( 'NONE',  ( -1.000000000000000000, 0.000000000000000000, 0.000000000000000000 ) ) ;
#17195=DIRECTION ( 'NONE',  ( -0.000000000000000000, -0.000000000000000000, 1.000000000000000000 ) ) ;
#17235=DIRECTION ( 'NONE',  ( 0.000000000000000000, 0.000000000000000000, -1.000000000000000000 ) ) ;
#17247=DIRECTION ( 'NONE',  ( -1.000000000000000000, 0.000000000000000000, 0.000000000000000000 ) ) ;
#17266=CARTESIAN_POINT ( 'NONE',  ( -62.49999999999997158, 32.50000000000001421, 15.00000000000000000 ) ) ;
#17275=CIRCLE ( 'NONE', #1303, 2.649999999999985700 ) ;
#17297=FACE_OUTER_BOUND ( 'NONE', #17892, .T. ) ;
#17308=VERTEX_POINT ( 'NONE', #11070 ) ;
#17325=DIRECTION ( 'NONE',  ( -1.000000000000000000, 0.000000000000000000, 0.000000000000000000 ) ) ;
#17348=ORIENTED_EDGE ( 'NONE', *, *, #18452, .T. ) ;
#17364=EDGE_CURVE ( 'NONE', #13076, #4248, #8480, .T. ) ;
#17365=ORIENTED_EDGE ( 'NONE', *, *, #1854, .T. ) ;
#17366=EDGE_CURVE ( 'NONE', #2192, #13670, #9985, .T. ) ;
#17392=DIRECTION ( 'NONE',  ( -1.000000000000000000, 0.000000000000000000, 0.000000000000000000 ) ) ;
#17441=EDGE_CURVE ( 'NONE', #3771, #15125, #5654, .T. ) ;
#17462=ORIENTED_EDGE ( 'NONE', *, *, #18278, .F. ) ;
#17466=AXIS2_PLACEMENT_3D ( 'NONE', #9031, #11771, #5903 ) ;
#17477=CARTESIAN_POINT ( 'NONE',  ( 62.49999999999998579, 40.00000000000001421, 0.000000000000000000 ) ) ;
#17492=DIRECTION ( 'NONE',  ( -1.000000000000000000, 0.000000000000000000, 0.000000000000000000 ) ) ;
#17496=EDGE_CURVE ( 'NONE', #17308, #6185, #13614, .T. ) ;
#17498=DIRECTION ( 'NONE',  ( 0.000000000000000000, 0.000000000000000000, -1.000000000000000000 ) ) ;
#17575=AXIS2_PLACEMENT_3D ( 'NONE', #16969, #3337, #7925 ) ;
#17590=VECTOR ( 'NONE', #17498, 1000.000000000000000 ) ;
#17621=CARTESIAN_POINT ( 'NONE',  ( 62.49999999999998579, 32.50000000000001421, -15.00000000000000000 ) ) ;
#17622=VECTOR ( 'NONE', #11531, 1000.000000000000000 ) ;
#17636=ORIENTED_EDGE ( 'NONE', *, *, #6302, .T. ) ;
#17675=EDGE_CURVE ( 'NONE', #9948, #6607, #18524, .T. ) ;
#17676=ADVANCED_FACE ( 'NONE', ( #674 ), #4893, .F. ) ;
#17678=VECTOR ( 'NONE', #17736, 1000.000000000000000 ) ;
#17689=CARTESIAN_POINT ( 'NONE',  ( 2.649999999999988809, 15.00000000000001599, -15.00000000000000000 ) ) ;
#17701=CARTESIAN_POINT ( 'NONE',  ( -74.99999999999997158, 45.00000000000001421, -15.00000000000000000 ) ) ;
#17702=VERTEX_POINT ( 'NONE', #5169 ) ;
#17704=CARTESIAN_POINT ( 'NONE',  ( -62.49999999999997158, 32.50000000000001421, 15.00000000000000000 ) ) ;
#17726=VECTOR ( 'NONE', #10974, 1000.000000000000000 ) ;
#17736=DIRECTION ( 'NONE',  ( -0.000000000000000000, -0.000000000000000000, -1.000000000000000000 ) ) ;
#17741=VERTEX_POINT ( 'NONE', #12184 ) ;
#17757=LINE ( 'NONE', #8824, #4587 ) ;
#17787=EDGE_CURVE ( 'NONE', #17949, #8729, #11087, .T. ) ;
#17816=ORIENTED_EDGE ( 'NONE', *, *, #2723, .T. ) ;
#17820=AXIS2_PLACEMENT_3D ( 'NONE', #6043, #1530, #4377 ) ;
#17823=ORIENTED_EDGE ( 'NONE', *, *, #3348, .F. ) ;
#17857=DIRECTION ( 'NONE',  ( -0.000000000000000000, -0.000000000000000000, 1.000000000000000000 ) ) ;
#17858=EDGE_CURVE ( 'NONE', #11648, #18236, #5025, .T. ) ;
#17863=VECTOR ( 'NONE', #8839, 1000.000000000000000 ) ;
#17868=( LENGTH_UNIT ( ) NAMED_UNIT ( * ) SI_UNIT ( .MILLI., .METRE. ) );
#17878=DIRECTION ( 'NONE',  ( 0.000000000000000000, 0.000000000000000000, -1.000000000000000000 ) ) ;
#17889=VERTEX_POINT ( 'NONE', #18476 ) ;
#17892=EDGE_LOOP ( 'NONE', ( #89, #16663, #5776, #11227 ) ) ;
#17913=PLANE ( 'NONE',  #15343 ) ;
#17926=AXIS2_PLACEMENT_3D ( 'NONE', #78, #4870, #12214 ) ;
#17948=DIRECTION ( 'NONE',  ( 0.000000000000000000, -0.000000000000000000, 1.000000000000000000 ) ) ;
#17949=VERTEX_POINT ( 'NONE', #5711 ) ;
#17987=ORIENTED_EDGE ( 'NONE', *, *, #14779, .F. ) ;
#17988=VECTOR ( 'NONE', #15542, 1000.000000000000000 ) ;
#17990=AXIS2_PLACEMENT_3D ( 'NONE', #11483, #6981, #17492 ) ;
#18019=ORIENTED_EDGE ( 'NONE', *, *, #10957, .F. ) ;
#18031=EDGE_CURVE ( 'NONE', #17889, #12519, #1012, .T. ) ;
#18062=EDGE_LOOP ( 'NONE', ( #17816, #3287, #15152, #14078 ) ) ;
#18064=SURFACE_STYLE_FILL_AREA ( #12344 ) ;
#18073=CARTESIAN_POINT ( 'NONE',  ( -9.999999999999998224, 15.00000000000001776, 9.999999999999998224 ) ) ;
#18090=ORIENTED_EDGE ( 'NONE', *, *, #11403, .F. ) ;
#18158=CARTESIAN_POINT ( 'NONE',  ( -9.999999999999996447, 0.000000000000000000, -9.999999999999998224 ) ) ;
#18198=LINE ( 'NONE', #7492, #2414 ) ;
#18209=CARTESIAN_POINT ( 'NONE',  ( 1.925929944387235853E-31, 15.00000000000001599, 15.00000000000000000 ) ) ;
#18215=LINE ( 'NONE', #7978, #16904 ) ;
#18221=ORIENTED_EDGE ( 'NONE', *, *, #19127, .T. ) ;
#18236=VERTEX_POINT ( 'NONE', #11033 ) ;
#18241=DIRECTION ( 'NONE',  ( 1.000000000000000000, 0.000000000000000000, 0.000000000000000000 ) ) ;
#18261=VECTOR ( 'NONE', #13135, 1000.000000000000000 ) ;
#18278=EDGE_CURVE ( 'NONE', #3771, #9070, #9656, .T. ) ;
#18280=EDGE_CURVE ( 'NONE', #11786, #6708, #13626, .T. ) ;
#18288=APPLICATION_CONTEXT ( 'automotive_design' ) ;
#18296=CARTESIAN_POINT ( 'NONE',  ( -62.49999999999997158, 32.50000000000001421, -9.999999999999998224 ) ) ;
#18355=SURFACE_STYLE_USAGE ( .BOTH. , #487 ) ;
#18357=( LENGTH_UNIT ( ) NAMED_UNIT ( * ) SI_UNIT ( .MILLI., .METRE. ) );
#18361=DIRECTION ( 'NONE',  ( -1.000000000000000000, 0.000000000000000000, 0.000000000000000000 ) ) ;
#18364=DIRECTION ( 'NONE',  ( -1.000000000000000000, 0.000000000000000000, 0.000000000000000000 ) ) ;
#18365=DIRECTION ( 'NONE',  ( -1.000000000000000000, 0.000000000000000000, 0.000000000000000000 ) ) ;
#18366=AXIS2_PLACEMENT_3D ( 'NONE', #970, #6840, #6651 ) ;
#18372=DIRECTION ( 'NONE',  ( 1.000000000000000000, 0.000000000000000000, 0.000000000000000000 ) ) ;
#18397=VECTOR ( 'NONE', #13272, 1000.000000000000000 ) ;
#18409=ORIENTED_EDGE ( 'NONE', *, *, #813, .F. ) ;
#18417=VECTOR ( 'NONE', #7032, 1000.000000000000000 ) ;
#18432=LINE ( 'NONE', #15770, #11595 ) ;
#18452=EDGE_CURVE ( 'NONE', #164, #7574, #12904, .T. ) ;
#18476=CARTESIAN_POINT ( 'NONE',  ( -2.649999999999988809, 15.00000000000001599, -15.00000000000000000 ) ) ;
#18517=AXIS2_PLACEMENT_3D ( 'NONE', #13839, #15410, #6478 ) ;
#18524=CIRCLE ( 'NONE', #10673, 12.49999999999999645 ) ;
#18528=FACE_OUTER_BOUND ( 'NONE', #15297, .T. ) ;
#18572=ADVANCED_FACE ( 'NONE', ( #16634, #12003, #4568 ), #17913, .T. ) ;
#18575=DIRECTION ( 'NONE',  ( 1.000000000000000000, 0.000000000000000000, 0.000000000000000000 ) ) ;
#18577=DIRECTION ( 'NONE',  ( 0.000000000000000000, -0.000000000000000000, 1.000000000000000000 ) ) ;
#18579=CARTESIAN_POINT ( 'NONE',  ( 62.49999999999998579, 45.00000000000001421, -5.000000000000000000 ) ) ;
#18585=CARTESIAN_POINT ( 'NONE',  ( -62.49999999999997158, 20.00000000000001421, 15.00000000000000000 ) ) ;
#18615=ORIENTED_EDGE ( 'NONE', *, *, #15885, .F. ) ;
#18638=EDGE_LOOP ( 'NONE', ( #397, #14143, #12780, #16871 ) ) ;
#18646=CARTESIAN_POINT ( 'NONE',  ( 10.00000000000000000, 15.00000000000001776, 9.999999999999998224 ) ) ;
#18649=CIRCLE ( 'NONE', #10166, 2.649999999999988809 ) ;
#18650=EDGE_LOOP ( 'NONE', ( #3989, #15551, #9776, #12643 ) ) ;
#18656=AXIS2_PLACEMENT_3D ( 'NONE', #17000, #12567, #18575 ) ;
#18674=LINE ( 'NONE', #5217, #7332 ) ;
#18693=ADVANCED_FACE ( 'NONE', ( #3381 ), #5131, .F. ) ;
#18699=EDGE_CURVE ( 'NONE', #5879, #17949, #3482, .T. ) ;
#18709=ORIENTED_EDGE ( 'NONE', *, *, #15134, .T. ) ;
#18730=ORIENTED_EDGE ( 'NONE', *, *, #2454, .T. ) ;
#18742=LINE ( 'NONE', #1349, #17622 ) ;
#18748=LINE ( 'NONE', #6858, #7563 ) ;
#18810=EDGE_LOOP ( 'NONE', ( #4139, #7557, #19078, #16324, #3993, #9125, #5065, #18019, #8566, #16248, #2358, #14251 ) ) ;
#18822=ORIENTED_EDGE ( 'NONE', *, *, #5122, .F. ) ;
#18826=VERTEX_POINT ( 'NONE', #5515 ) ;
#18835=AXIS2_PLACEMENT_3D ( 'NONE', #4083, #14164, #3796 ) ;
#18865=AXIS2_PLACEMENT_3D ( 'NONE', #14332, #916, #7183 ) ;
#18872=FACE_BOUND ( 'NONE', #854, .T. ) ;
#18884=ORIENTED_EDGE ( 'NONE', *, *, #17787, .F. ) ;
#18915=ORIENTED_EDGE ( 'NONE', *, *, #3055, .T. ) ;
#18919=FACE_OUTER_BOUND ( 'NONE', #11527, .T. ) ;
#18936=CARTESIAN_POINT ( 'NONE',  ( 2.649999999999988365, 15.00000000000001599, 15.00000000000000000 ) ) ;
#18983=CARTESIAN_POINT ( 'NONE',  ( 62.49999999999998579, 32.50000000000001421, 15.00000000000000000 ) ) ;
#19005=EDGE_LOOP ( 'NONE', ( #5079, #4816, #11784, #1027 ) ) ;
#19016=ORIENTED_EDGE ( 'NONE', *, *, #4237, .F. ) ;
#19020=DIRECTION ( 'NONE',  ( 0.000000000000000000, 0.000000000000000000, -1.000000000000000000 ) ) ;
#19025=CARTESIAN_POINT ( 'NONE',  ( 62.49999999999998579, 5.000000000000018652, 5.000000000000000000 ) ) ;
#19029=ORIENTED_EDGE ( 'NONE', *, *, #7417, .T. ) ;
#19078=ORIENTED_EDGE ( 'NONE', *, *, #14355, .F. ) ;
#19087=CIRCLE ( 'NONE', #8405, 12.49999999999999645 ) ;
#19088=VERTEX_POINT ( 'NONE', #7286 ) ;
#19090=EDGE_LOOP ( 'NONE', ( #5840, #8498, #4502, #18221 ) ) ;
#19095=DIRECTION ( 'NONE',  ( -1.000000000000000000, 0.000000000000000000, 0.000000000000000000 ) ) ;
#19105=ORIENTED_EDGE ( 'NONE', *, *, #14050, .T. ) ;
#19123=LINE ( 'NONE', #1353, #9853 ) ;
#19124=VECTOR ( 'NONE', #4715, 1000.000000000000000 ) ;
#19127=EDGE_CURVE ( 'NONE', #17949, #2897, #16508, .T. ) ;
#19172=CARTESIAN_POINT ( 'NONE',  ( -65.14999999999996305, 32.50000000000001421, 9.999999999999998224 ) ) ;
#19186=ORIENTED_EDGE ( 'NONE', *, *, #12800, .T. ) ;
#19237=CARTESIAN_POINT ( 'NONE',  ( 1.925929944387235853E-31, 15.00000000000001599, 15.00000000000000178 ) ) ;
#19279=ORIENTED_EDGE ( 'NONE', *, *, #14173, .T. ) ;
#19312=ADVANCED_FACE ( 'NONE', ( #4644 ), #16608, .T. ) ;
#19322=DIRECTION ( 'NONE',  ( -0.000000000000000000, 1.000000000000000000, -0.000000000000000000 ) ) ;
#19332=VECTOR ( 'NONE', #5885, 1000.000000000000000 ) ;
#19338=DIRECTION ( 'NONE',  ( -1.000000000000000000, 0.000000000000000000, 0.000000000000000000 ) ) ;
#19382=ORIENTED_EDGE ( 'NONE', *, *, #6502, .T. ) ;
#19394=AXIS2_PLACEMENT_3D ( 'NONE', #16465, #7626, #3509 ) ;
#19455=COLOUR_RGB('Sky Blue',0.24,0.69,0.87);
#19456=FILL_AREA_STYLE_COLOUR('',#19455);
#19457=FILL_AREA_STYLE('',(#19456));
#19458=SURFACE_STYLE_FILL_AREA(#19457);
#19459=SURFACE_SIDE_STYLE('',(#19458));
#19460=SURFACE_STYLE_USAGE(.BOTH.,#19459);
#19461=PRESENTATION_STYLE_ASSIGNMENT((#19460));
ENDSEC;
END-ISO-10303-21;
